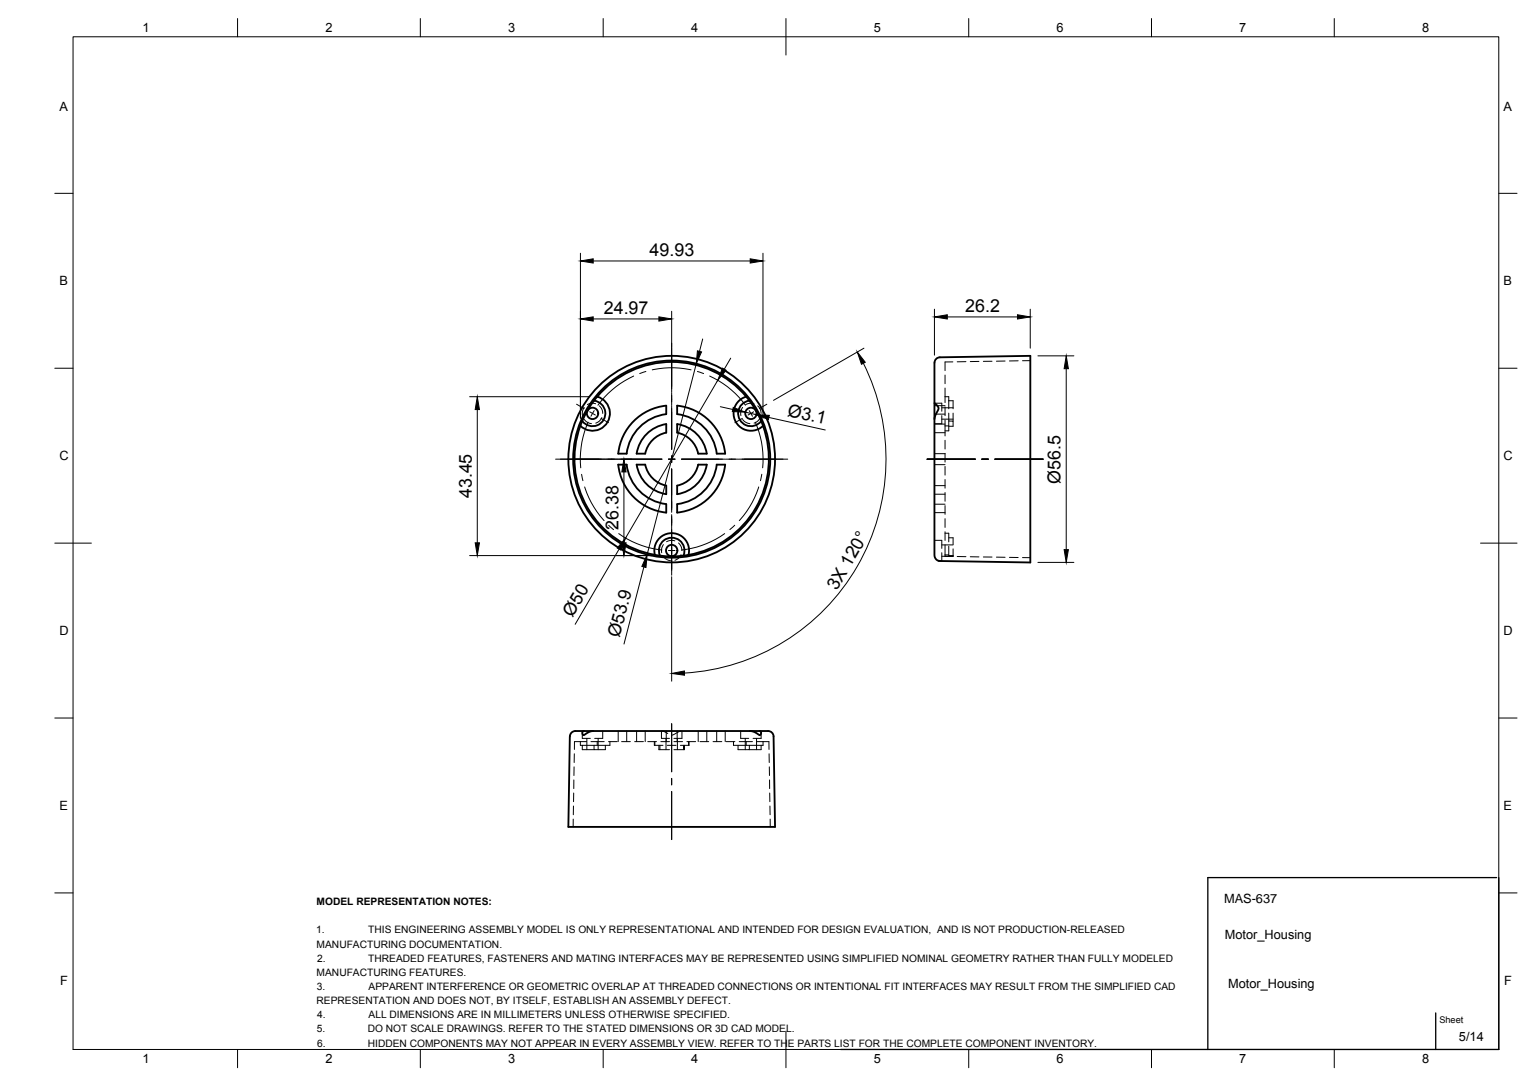
ISO-10303-21;
HEADER;
FILE_DESCRIPTION((''),'2;1');
FILE_NAME('Motor_Housing.step','2026-10-09T10:11:57-07:00',(''),(''),'','','');
FILE_SCHEMA (('AUTOMOTIVE_DESIGN { 1 0 10303 214 3 1 1 }'));
ENDSEC;
DATA;
#10=MECHANICAL_DESIGN_GEOMETRIC_PRESENTATION_REPRESENTATION('',(#125),#13510);
#95=SHAPE_REPRESENTATION_RELATIONSHIP('SRR','None',#13565,#110) ;
#110=ADVANCED_BREP_SHAPE_REPRESENTATION('',(#157),#13497) ;
#125=STYLED_ITEM('',(#13649),#157) ;
#157=MANIFOLD_SOLID_BREP('Body1',#7374) ;
#217=FACE_BOUND('',#1283,.T.) ;
#218=FACE_BOUND('',#1286,.T.) ;
#219=FACE_BOUND('',#1292,.T.) ;
#220=FACE_BOUND('',#1335,.T.) ;
#221=FACE_BOUND('',#1336,.T.) ;
#222=FACE_BOUND('',#1337,.T.) ;
#223=FACE_BOUND('',#1338,.T.) ;
#224=FACE_BOUND('',#1339,.T.) ;
#225=FACE_BOUND('',#1340,.T.) ;
#226=FACE_BOUND('',#1341,.T.) ;
#227=FACE_BOUND('',#1342,.T.) ;
#228=FACE_BOUND('',#1346,.T.) ;
#229=FACE_BOUND('',#1348,.T.) ;
#230=FACE_BOUND('',#1350,.T.) ;
#231=FACE_BOUND('',#1351,.T.) ;
#232=FACE_BOUND('',#1352,.T.) ;
#233=FACE_BOUND('',#1353,.T.) ;
#234=FACE_BOUND('',#1354,.T.) ;
#235=FACE_BOUND('',#1355,.T.) ;
#236=FACE_BOUND('',#1356,.T.) ;
#237=FACE_BOUND('',#1357,.T.) ;
#238=FACE_BOUND('',#1360,.T.) ;
#239=FACE_BOUND('',#1364,.T.) ;
#324=PLANE('',#7894) ;
#325=PLANE('',#7899) ;
#326=PLANE('',#7919) ;
#327=PLANE('',#7929) ;
#328=PLANE('',#7933) ;
#329=PLANE('',#7944) ;
#330=PLANE('',#7948) ;
#331=PLANE('',#7952) ;
#332=PLANE('',#7956) ;
#333=PLANE('',#7960) ;
#334=PLANE('',#7964) ;
#335=PLANE('',#7965) ;
#336=PLANE('',#7969) ;
#337=PLANE('',#7973) ;
#338=PLANE('',#7977) ;
#339=PLANE('',#7981) ;
#340=PLANE('',#7985) ;
#341=PLANE('',#7989) ;
#342=PLANE('',#7993) ;
#343=PLANE('',#7997) ;
#344=PLANE('',#8001) ;
#345=PLANE('',#8009) ;
#346=PLANE('',#8010) ;
#347=PLANE('',#8014) ;
#348=PLANE('',#8016) ;
#349=PLANE('',#8018) ;
#350=PLANE('',#8029) ;
#351=PLANE('',#8034) ;
#489=B_SPLINE_CURVE_WITH_KNOTS('',3,(#12264,#12265,#12266,#12267,#12268,
#12269,#12270,#12271,#12272,#12273,#12274,#12275,#12276,#12277,#12278,#12279,
#12280,#12281,#12282,#12283,#12284,#12285,#12286,#12287,#12288,#12289,#12290,
#12291,#12292,#12293,#12294,#12295,#12296,#12297),.UNSPECIFIED.,.F.,.F.,
(4,2,2,2,2,2,2,2,2,2,2,2,2,2,2,2,4),(0.531805899879346,0.536333824755711,
0.591897384336284,0.667209604638838,0.739839654066166,0.796834727976756,
0.805195853248504,0.808326840958196,0.810223650281403,0.812270988818894,
0.815029287812512,0.821153230725477,0.854786642673204,0.894100597636804,
0.968451976824404,1.02522403229621,1.04311608969068),.UNSPECIFIED.) ;
#490=B_SPLINE_CURVE_WITH_KNOTS('',3,(#12324,#12325,#12326,#12327,#12328,
#12329,#12330,#12331,#12332,#12333,#12334,#12335,#12336,#12337,#12338,#12339,
#12340,#12341,#12342,#12343,#12344,#12345,#12346,#12347,#12348,#12349,#12350,
#12351,#12352,#12353,#12354,#12355,#12356,#12357),.UNSPECIFIED.,.F.,.F.,
(4,2,2,2,2,2,2,2,2,2,2,2,2,2,2,2,4),(-1.04311608843254,-1.02522403109388,
-0.968451975747413,-0.894100596714524,-0.854786641825103,-0.821153229937673,
-0.815029287031212,-0.812270988041687,-0.810223649507742,-0.808326840188323,
-0.805195852486152,-0.796834727237095,-0.739839653424281,-0.667209604095289,
-0.591897383884855,-0.536333824369451,-0.531805899490485),.UNSPECIFIED.) ;
#491=B_SPLINE_CURVE_WITH_KNOTS('',3,(#12358,#12359,#12360,#12361,#12362,
#12363,#12364,#12365,#12366,#12367,#12368,#12369,#12370,#12371,#12372,#12373,
#12374,#12375,#12376,#12377,#12378,#12379,#12380,#12381,#12382,#12383,#12384,
#12385,#12386,#12387,#12388,#12389,#12390,#12391),.UNSPECIFIED.,.F.,.F.,
(4,2,2,2,2,2,2,2,2,2,2,2,2,2,2,2,4),(-1.04311608859891,-1.02522403125026,
-0.968451975875515,-0.8941005968091,-0.854786641903559,-0.821153230003261,
-0.815029287094133,-0.812270988104498,-0.8102236495713,-0.808326840252012,
-0.805195852547876,-0.796834727295025,-0.73983965345829,-0.667209604102352,
-0.59189738386758,-0.53633382433688,-0.531805899459014),.UNSPECIFIED.) ;
#497=TOROIDAL_SURFACE('',#8027,26.3501962679,1.5) ;
#601=CYLINDRICAL_SURFACE('',#7897,1.55) ;
#602=CYLINDRICAL_SURFACE('',#7902,26.5728722547) ;
#603=CYLINDRICAL_SURFACE('',#7906,3.5) ;
#604=CYLINDRICAL_SURFACE('',#7916,4.75) ;
#605=CYLINDRICAL_SURFACE('',#7923,3.5) ;
#606=CYLINDRICAL_SURFACE('',#7926,3.5) ;
#607=CYLINDRICAL_SURFACE('',#7937,4.75) ;
#608=CYLINDRICAL_SURFACE('',#7939,4.75) ;
#609=CYLINDRICAL_SURFACE('',#7941,12.4) ;
#610=CYLINDRICAL_SURFACE('',#7945,14.7) ;
#611=CYLINDRICAL_SURFACE('',#7949,7.4) ;
#612=CYLINDRICAL_SURFACE('',#7953,9.7) ;
#613=CYLINDRICAL_SURFACE('',#7957,12.4) ;
#614=CYLINDRICAL_SURFACE('',#7961,14.7) ;
#615=CYLINDRICAL_SURFACE('',#7966,12.4) ;
#616=CYLINDRICAL_SURFACE('',#7970,14.7) ;
#617=CYLINDRICAL_SURFACE('',#7974,9.7) ;
#618=CYLINDRICAL_SURFACE('',#7978,7.4) ;
#619=CYLINDRICAL_SURFACE('',#7982,9.7) ;
#620=CYLINDRICAL_SURFACE('',#7986,7.4) ;
#621=CYLINDRICAL_SURFACE('',#7990,7.4) ;
#622=CYLINDRICAL_SURFACE('',#7994,9.7) ;
#623=CYLINDRICAL_SURFACE('',#7998,14.7) ;
#624=CYLINDRICAL_SURFACE('',#8002,12.4) ;
#625=CYLINDRICAL_SURFACE('',#8005,26.5728722547) ;
#626=CYLINDRICAL_SURFACE('',#8007,26.5728722547) ;
#627=CYLINDRICAL_SURFACE('',#8011,2.8) ;
#628=CYLINDRICAL_SURFACE('',#8032,2.8) ;
#629=CYLINDRICAL_SURFACE('',#8033,1.55) ;
#630=CYLINDRICAL_SURFACE('',#8037,2.8) ;
#631=CYLINDRICAL_SURFACE('',#8038,1.55) ;
#804=FACE_OUTER_BOUND('',#1282,.T.) ;
#805=FACE_OUTER_BOUND('',#1284,.T.) ;
#806=FACE_OUTER_BOUND('',#1285,.T.) ;
#807=FACE_OUTER_BOUND('',#1287,.T.) ;
#808=FACE_OUTER_BOUND('',#1288,.T.) ;
#809=FACE_OUTER_BOUND('',#1289,.T.) ;
#810=FACE_OUTER_BOUND('',#1290,.T.) ;
#811=FACE_OUTER_BOUND('',#1291,.T.) ;
#812=FACE_OUTER_BOUND('',#1293,.T.) ;
#813=FACE_OUTER_BOUND('',#1294,.T.) ;
#814=FACE_OUTER_BOUND('',#1295,.T.) ;
#815=FACE_OUTER_BOUND('',#1296,.T.) ;
#816=FACE_OUTER_BOUND('',#1297,.T.) ;
#817=FACE_OUTER_BOUND('',#1298,.T.) ;
#818=FACE_OUTER_BOUND('',#1299,.T.) ;
#819=FACE_OUTER_BOUND('',#1300,.T.) ;
#820=FACE_OUTER_BOUND('',#1301,.T.) ;
#821=FACE_OUTER_BOUND('',#1302,.T.) ;
#822=FACE_OUTER_BOUND('',#1303,.T.) ;
#823=FACE_OUTER_BOUND('',#1304,.T.) ;
#824=FACE_OUTER_BOUND('',#1305,.T.) ;
#825=FACE_OUTER_BOUND('',#1306,.T.) ;
#826=FACE_OUTER_BOUND('',#1307,.T.) ;
#827=FACE_OUTER_BOUND('',#1308,.T.) ;
#828=FACE_OUTER_BOUND('',#1309,.T.) ;
#829=FACE_OUTER_BOUND('',#1310,.T.) ;
#830=FACE_OUTER_BOUND('',#1311,.T.) ;
#831=FACE_OUTER_BOUND('',#1312,.T.) ;
#832=FACE_OUTER_BOUND('',#1313,.T.) ;
#833=FACE_OUTER_BOUND('',#1314,.T.) ;
#834=FACE_OUTER_BOUND('',#1315,.T.) ;
#835=FACE_OUTER_BOUND('',#1316,.T.) ;
#836=FACE_OUTER_BOUND('',#1317,.T.) ;
#837=FACE_OUTER_BOUND('',#1318,.T.) ;
#838=FACE_OUTER_BOUND('',#1319,.T.) ;
#839=FACE_OUTER_BOUND('',#1320,.T.) ;
#840=FACE_OUTER_BOUND('',#1321,.T.) ;
#841=FACE_OUTER_BOUND('',#1322,.T.) ;
#842=FACE_OUTER_BOUND('',#1323,.T.) ;
#843=FACE_OUTER_BOUND('',#1324,.T.) ;
#844=FACE_OUTER_BOUND('',#1325,.T.) ;
#845=FACE_OUTER_BOUND('',#1326,.T.) ;
#846=FACE_OUTER_BOUND('',#1327,.T.) ;
#847=FACE_OUTER_BOUND('',#1328,.T.) ;
#848=FACE_OUTER_BOUND('',#1329,.T.) ;
#849=FACE_OUTER_BOUND('',#1330,.T.) ;
#850=FACE_OUTER_BOUND('',#1331,.T.) ;
#851=FACE_OUTER_BOUND('',#1332,.T.) ;
#852=FACE_OUTER_BOUND('',#1333,.T.) ;
#853=FACE_OUTER_BOUND('',#1334,.T.) ;
#854=FACE_OUTER_BOUND('',#1343,.T.) ;
#855=FACE_OUTER_BOUND('',#1344,.T.) ;
#856=FACE_OUTER_BOUND('',#1345,.T.) ;
#857=FACE_OUTER_BOUND('',#1347,.T.) ;
#858=FACE_OUTER_BOUND('',#1349,.T.) ;
#859=FACE_OUTER_BOUND('',#1358,.T.) ;
#860=FACE_OUTER_BOUND('',#1359,.T.) ;
#861=FACE_OUTER_BOUND('',#1361,.T.) ;
#862=FACE_OUTER_BOUND('',#1362,.T.) ;
#863=FACE_OUTER_BOUND('',#1363,.T.) ;
#864=FACE_OUTER_BOUND('',#1365,.T.) ;
#865=FACE_OUTER_BOUND('',#1366,.T.) ;
#1282=EDGE_LOOP('',(#5566)) ;
#1283=EDGE_LOOP('',(#5567)) ;
#1284=EDGE_LOOP('',(#5568,#5569,#5570,#5571)) ;
#1285=EDGE_LOOP('',(#5572,#5573)) ;
#1286=EDGE_LOOP('',(#5574)) ;
#1287=EDGE_LOOP('',(#5575,#5576,#5577,#5578,#5579,#5580,#5581,#5582)) ;
#1288=EDGE_LOOP('',(#5583,#5584,#5585,#5586)) ;
#1289=EDGE_LOOP('',(#5587,#5588,#5589,#5590,#5591,#5592,#5593,#5594,#5595,
#5596)) ;
#1290=EDGE_LOOP('',(#5597,#5598,#5599,#5600)) ;
#1291=EDGE_LOOP('',(#5601)) ;
#1292=EDGE_LOOP('',(#5602)) ;
#1293=EDGE_LOOP('',(#5603,#5604,#5605,#5606)) ;
#1294=EDGE_LOOP('',(#5607,#5608,#5609,#5610)) ;
#1295=EDGE_LOOP('',(#5611,#5612,#5613,#5614)) ;
#1296=EDGE_LOOP('',(#5615,#5616,#5617,#5618)) ;
#1297=EDGE_LOOP('',(#5619,#5620,#5621,#5622)) ;
#1298=EDGE_LOOP('',(#5623,#5624,#5625,#5626)) ;
#1299=EDGE_LOOP('',(#5627,#5628,#5629,#5630)) ;
#1300=EDGE_LOOP('',(#5631,#5632,#5633,#5634)) ;
#1301=EDGE_LOOP('',(#5635,#5636,#5637,#5638)) ;
#1302=EDGE_LOOP('',(#5639,#5640,#5641,#5642)) ;
#1303=EDGE_LOOP('',(#5643,#5644,#5645,#5646)) ;
#1304=EDGE_LOOP('',(#5647,#5648,#5649,#5650)) ;
#1305=EDGE_LOOP('',(#5651,#5652,#5653,#5654)) ;
#1306=EDGE_LOOP('',(#5655,#5656,#5657,#5658)) ;
#1307=EDGE_LOOP('',(#5659,#5660,#5661,#5662)) ;
#1308=EDGE_LOOP('',(#5663,#5664,#5665,#5666)) ;
#1309=EDGE_LOOP('',(#5667,#5668,#5669,#5670)) ;
#1310=EDGE_LOOP('',(#5671,#5672,#5673,#5674)) ;
#1311=EDGE_LOOP('',(#5675,#5676,#5677,#5678)) ;
#1312=EDGE_LOOP('',(#5679,#5680,#5681,#5682)) ;
#1313=EDGE_LOOP('',(#5683,#5684,#5685,#5686)) ;
#1314=EDGE_LOOP('',(#5687,#5688,#5689,#5690)) ;
#1315=EDGE_LOOP('',(#5691,#5692,#5693,#5694)) ;
#1316=EDGE_LOOP('',(#5695,#5696,#5697,#5698)) ;
#1317=EDGE_LOOP('',(#5699,#5700,#5701,#5702)) ;
#1318=EDGE_LOOP('',(#5703,#5704,#5705,#5706)) ;
#1319=EDGE_LOOP('',(#5707,#5708,#5709,#5710)) ;
#1320=EDGE_LOOP('',(#5711,#5712,#5713,#5714)) ;
#1321=EDGE_LOOP('',(#5715,#5716,#5717,#5718)) ;
#1322=EDGE_LOOP('',(#5719,#5720,#5721,#5722)) ;
#1323=EDGE_LOOP('',(#5723,#5724,#5725,#5726)) ;
#1324=EDGE_LOOP('',(#5727,#5728,#5729,#5730)) ;
#1325=EDGE_LOOP('',(#5731,#5732,#5733,#5734)) ;
#1326=EDGE_LOOP('',(#5735,#5736,#5737,#5738)) ;
#1327=EDGE_LOOP('',(#5739,#5740,#5741,#5742)) ;
#1328=EDGE_LOOP('',(#5743,#5744,#5745,#5746)) ;
#1329=EDGE_LOOP('',(#5747,#5748,#5749,#5750)) ;
#1330=EDGE_LOOP('',(#5751,#5752,#5753,#5754)) ;
#1331=EDGE_LOOP('',(#5755,#5756,#5757,#5758)) ;
#1332=EDGE_LOOP('',(#5759,#5760,#5761,#5762,#5763,#5764,#5765,#5766)) ;
#1333=EDGE_LOOP('',(#5767,#5768,#5769,#5770,#5771,#5772,#5773,#5774)) ;
#1334=EDGE_LOOP('',(#5775,#5776,#5777,#5778,#5779,#5780,#5781)) ;
#1335=EDGE_LOOP('',(#5782,#5783,#5784,#5785)) ;
#1336=EDGE_LOOP('',(#5786,#5787,#5788,#5789)) ;
#1337=EDGE_LOOP('',(#5790,#5791,#5792,#5793)) ;
#1338=EDGE_LOOP('',(#5794,#5795,#5796,#5797)) ;
#1339=EDGE_LOOP('',(#5798,#5799,#5800,#5801)) ;
#1340=EDGE_LOOP('',(#5802,#5803,#5804,#5805)) ;
#1341=EDGE_LOOP('',(#5806,#5807,#5808,#5809)) ;
#1342=EDGE_LOOP('',(#5810,#5811,#5812,#5813)) ;
#1343=EDGE_LOOP('',(#5814,#5815,#5816,#5817)) ;
#1344=EDGE_LOOP('',(#5818,#5819,#5820,#5821,#5822,#5823)) ;
#1345=EDGE_LOOP('',(#5824,#5825)) ;
#1346=EDGE_LOOP('',(#5826)) ;
#1347=EDGE_LOOP('',(#5827,#5828)) ;
#1348=EDGE_LOOP('',(#5829)) ;
#1349=EDGE_LOOP('',(#5830,#5831,#5832,#5833,#5834,#5835,#5836,#5837,#5838,
#5839)) ;
#1350=EDGE_LOOP('',(#5840,#5841,#5842,#5843)) ;
#1351=EDGE_LOOP('',(#5844,#5845,#5846,#5847)) ;
#1352=EDGE_LOOP('',(#5848,#5849,#5850,#5851)) ;
#1353=EDGE_LOOP('',(#5852,#5853,#5854,#5855)) ;
#1354=EDGE_LOOP('',(#5856,#5857,#5858,#5859)) ;
#1355=EDGE_LOOP('',(#5860,#5861,#5862,#5863)) ;
#1356=EDGE_LOOP('',(#5864,#5865,#5866,#5867)) ;
#1357=EDGE_LOOP('',(#5868,#5869,#5870,#5871)) ;
#1358=EDGE_LOOP('',(#5872,#5873,#5874,#5875,#5876,#5877,#5878,#5879,#5880,
#5881)) ;
#1359=EDGE_LOOP('',(#5882)) ;
#1360=EDGE_LOOP('',(#5883)) ;
#1361=EDGE_LOOP('',(#5884,#5885,#5886,#5887,#5888,#5889)) ;
#1362=EDGE_LOOP('',(#5890,#5891,#5892,#5893)) ;
#1363=EDGE_LOOP('',(#5894)) ;
#1364=EDGE_LOOP('',(#5895)) ;
#1365=EDGE_LOOP('',(#5896,#5897,#5898,#5899,#5900,#5901)) ;
#1366=EDGE_LOOP('',(#5902,#5903,#5904,#5905)) ;
#1822=LINE('',#11975,#2316) ;
#1823=LINE('',#11987,#2317) ;
#1824=LINE('',#11990,#2318) ;
#1825=LINE('',#11992,#2319) ;
#1826=LINE('',#11995,#2320) ;
#1827=LINE('',#12011,#2321) ;
#1828=LINE('',#12021,#2322) ;
#1829=LINE('',#12026,#2323) ;
#1830=LINE('',#12030,#2324) ;
#1831=LINE('',#12035,#2325) ;
#1832=LINE('',#12039,#2326) ;
#1833=LINE('',#12054,#2327) ;
#1834=LINE('',#12056,#2328) ;
#1835=LINE('',#12058,#2329) ;
#1836=LINE('',#12060,#2330) ;
#1837=LINE('',#12064,#2331) ;
#1838=LINE('',#12068,#2332) ;
#1839=LINE('',#12072,#2333) ;
#1840=LINE('',#12074,#2334) ;
#1841=LINE('',#12075,#2335) ;
#1842=LINE('',#12080,#2336) ;
#1843=LINE('',#12083,#2337) ;
#1844=LINE('',#12084,#2338) ;
#1845=LINE('',#12088,#2339) ;
#1846=LINE('',#12092,#2340) ;
#1847=LINE('',#12096,#2341) ;
#1848=LINE('',#12098,#2342) ;
#1849=LINE('',#12099,#2343) ;
#1850=LINE('',#12104,#2344) ;
#1851=LINE('',#12107,#2345) ;
#1852=LINE('',#12108,#2346) ;
#1853=LINE('',#12112,#2347) ;
#1854=LINE('',#12116,#2348) ;
#1855=LINE('',#12121,#2349) ;
#1856=LINE('',#12122,#2350) ;
#1857=LINE('',#12123,#2351) ;
#1858=LINE('',#12128,#2352) ;
#1859=LINE('',#12131,#2353) ;
#1860=LINE('',#12132,#2354) ;
#1861=LINE('',#12136,#2355) ;
#1862=LINE('',#12138,#2356) ;
#1863=LINE('',#12140,#2357) ;
#1864=LINE('',#12141,#2358) ;
#1865=LINE('',#12145,#2359) ;
#1866=LINE('',#12151,#2360) ;
#1867=LINE('',#12152,#2361) ;
#1868=LINE('',#12153,#2362) ;
#1869=LINE('',#12160,#2363) ;
#1870=LINE('',#12162,#2364) ;
#1871=LINE('',#12164,#2365) ;
#1872=LINE('',#12165,#2366) ;
#1873=LINE('',#12170,#2367) ;
#1874=LINE('',#12175,#2368) ;
#1875=LINE('',#12176,#2369) ;
#1876=LINE('',#12177,#2370) ;
#1877=LINE('',#12184,#2371) ;
#1878=LINE('',#12186,#2372) ;
#1879=LINE('',#12188,#2373) ;
#1880=LINE('',#12189,#2374) ;
#1881=LINE('',#12194,#2375) ;
#1882=LINE('',#12199,#2376) ;
#1883=LINE('',#12200,#2377) ;
#1884=LINE('',#12201,#2378) ;
#1885=LINE('',#12208,#2379) ;
#1886=LINE('',#12210,#2380) ;
#1887=LINE('',#12212,#2381) ;
#1888=LINE('',#12213,#2382) ;
#1889=LINE('',#12217,#2383) ;
#1890=LINE('',#12223,#2384) ;
#1891=LINE('',#12224,#2385) ;
#1892=LINE('',#12225,#2386) ;
#1893=LINE('',#12232,#2387) ;
#1894=LINE('',#12234,#2388) ;
#1895=LINE('',#12236,#2389) ;
#1896=LINE('',#12237,#2390) ;
#1897=LINE('',#12242,#2391) ;
#1898=LINE('',#12247,#2392) ;
#1899=LINE('',#12248,#2393) ;
#1900=LINE('',#12249,#2394) ;
#1901=LINE('',#12299,#2395) ;
#1902=LINE('',#12398,#2396) ;
#1903=LINE('',#12400,#2397) ;
#1904=LINE('',#12407,#2398) ;
#1905=LINE('',#12409,#2399) ;
#2316=VECTOR('',#9396,1.55) ;
#2317=VECTOR('',#9409,1.) ;
#2318=VECTOR('',#9412,1.) ;
#2319=VECTOR('',#9413,1.) ;
#2320=VECTOR('',#9416,1.) ;
#2321=VECTOR('',#9435,26.5728722547) ;
#2322=VECTOR('',#9450,27.85) ;
#2323=VECTOR('',#9455,1.) ;
#2324=VECTOR('',#9458,1.) ;
#2325=VECTOR('',#9463,1.) ;
#2326=VECTOR('',#9466,1.) ;
#2327=VECTOR('',#9487,1.) ;
#2328=VECTOR('',#9490,1.) ;
#2329=VECTOR('',#9493,1.) ;
#2330=VECTOR('',#9496,1.) ;
#2331=VECTOR('',#9499,1.) ;
#2332=VECTOR('',#9502,1.) ;
#2333=VECTOR('',#9507,1.) ;
#2334=VECTOR('',#9508,1.) ;
#2335=VECTOR('',#9509,1.) ;
#2336=VECTOR('',#9514,1.) ;
#2337=VECTOR('',#9519,1.) ;
#2338=VECTOR('',#9520,1.) ;
#2339=VECTOR('',#9523,1.) ;
#2340=VECTOR('',#9526,1.) ;
#2341=VECTOR('',#9531,1.) ;
#2342=VECTOR('',#9532,1.) ;
#2343=VECTOR('',#9533,1.) ;
#2344=VECTOR('',#9538,1.) ;
#2345=VECTOR('',#9543,1.) ;
#2346=VECTOR('',#9544,1.) ;
#2347=VECTOR('',#9547,1.) ;
#2348=VECTOR('',#9550,1.) ;
#2349=VECTOR('',#9555,1.) ;
#2350=VECTOR('',#9556,1.) ;
#2351=VECTOR('',#9557,1.) ;
#2352=VECTOR('',#9562,1.) ;
#2353=VECTOR('',#9567,1.) ;
#2354=VECTOR('',#9568,1.) ;
#2355=VECTOR('',#9571,1.) ;
#2356=VECTOR('',#9572,1.) ;
#2357=VECTOR('',#9573,1.) ;
#2358=VECTOR('',#9574,1.) ;
#2359=VECTOR('',#9577,1.) ;
#2360=VECTOR('',#9584,1.) ;
#2361=VECTOR('',#9585,1.) ;
#2362=VECTOR('',#9586,1.) ;
#2363=VECTOR('',#9595,1.) ;
#2364=VECTOR('',#9596,1.) ;
#2365=VECTOR('',#9597,1.) ;
#2366=VECTOR('',#9598,1.) ;
#2367=VECTOR('',#9603,1.) ;
#2368=VECTOR('',#9608,1.) ;
#2369=VECTOR('',#9609,1.) ;
#2370=VECTOR('',#9610,1.) ;
#2371=VECTOR('',#9619,1.) ;
#2372=VECTOR('',#9620,1.) ;
#2373=VECTOR('',#9621,1.) ;
#2374=VECTOR('',#9622,1.) ;
#2375=VECTOR('',#9627,1.) ;
#2376=VECTOR('',#9632,1.) ;
#2377=VECTOR('',#9633,1.) ;
#2378=VECTOR('',#9634,1.) ;
#2379=VECTOR('',#9643,1.) ;
#2380=VECTOR('',#9644,1.) ;
#2381=VECTOR('',#9645,1.) ;
#2382=VECTOR('',#9646,1.) ;
#2383=VECTOR('',#9649,1.) ;
#2384=VECTOR('',#9656,1.) ;
#2385=VECTOR('',#9657,1.) ;
#2386=VECTOR('',#9658,1.) ;
#2387=VECTOR('',#9667,1.) ;
#2388=VECTOR('',#9668,1.) ;
#2389=VECTOR('',#9669,1.) ;
#2390=VECTOR('',#9670,1.) ;
#2391=VECTOR('',#9675,1.) ;
#2392=VECTOR('',#9680,1.) ;
#2393=VECTOR('',#9681,1.) ;
#2394=VECTOR('',#9682,1.) ;
#2395=VECTOR('',#9707,2.8) ;
#2396=VECTOR('',#9746,2.8) ;
#2397=VECTOR('',#9749,1.55) ;
#2398=VECTOR('',#9758,2.8) ;
#2399=VECTOR('',#9761,1.55) ;
#2815=CIRCLE('',#7895,2.8) ;
#2816=CIRCLE('',#7896,1.55) ;
#2817=CIRCLE('',#7898,1.55) ;
#2818=CIRCLE('',#7900,26.5728722547) ;
#2819=CIRCLE('',#7901,3.5) ;
#2820=CIRCLE('',#7903,26.5728722547) ;
#2821=CIRCLE('',#7904,26.5728722547) ;
#2822=CIRCLE('',#7905,26.5728722547) ;
#2823=CIRCLE('',#7907,3.5) ;
#2824=CIRCLE('',#7909,26.5728722547) ;
#2825=CIRCLE('',#7910,26.5728722547) ;
#2826=CIRCLE('',#7911,26.5728722547) ;
#2827=CIRCLE('',#7912,26.5728722547) ;
#2828=CIRCLE('',#7913,26.5728722547) ;
#2829=CIRCLE('',#7914,26.5728722547) ;
#2830=CIRCLE('',#7915,26.9498298789) ;
#2831=CIRCLE('',#7917,4.75) ;
#2832=CIRCLE('',#7918,4.75) ;
#2833=CIRCLE('',#7920,28.25) ;
#2834=CIRCLE('',#7922,27.85) ;
#2835=CIRCLE('',#7924,3.5) ;
#2836=CIRCLE('',#7925,3.5) ;
#2837=CIRCLE('',#7927,3.5) ;
#2838=CIRCLE('',#7928,3.5) ;
#2839=CIRCLE('',#7930,26.5728722547) ;
#2840=CIRCLE('',#7931,4.75) ;
#2841=CIRCLE('',#7932,26.5728722547) ;
#2842=CIRCLE('',#7934,26.5728722547) ;
#2843=CIRCLE('',#7935,4.75) ;
#2844=CIRCLE('',#7936,26.5728722547) ;
#2845=CIRCLE('',#7938,4.75) ;
#2846=CIRCLE('',#7940,4.75) ;
#2847=CIRCLE('',#7942,12.4) ;
#2848=CIRCLE('',#7943,12.4) ;
#2849=CIRCLE('',#7946,14.7) ;
#2850=CIRCLE('',#7947,14.7) ;
#2851=CIRCLE('',#7950,7.4) ;
#2852=CIRCLE('',#7951,7.4) ;
#2853=CIRCLE('',#7954,9.7) ;
#2854=CIRCLE('',#7955,9.7) ;
#2855=CIRCLE('',#7958,12.4) ;
#2856=CIRCLE('',#7959,12.4) ;
#2857=CIRCLE('',#7962,14.7) ;
#2858=CIRCLE('',#7963,14.7) ;
#2859=CIRCLE('',#7967,12.4) ;
#2860=CIRCLE('',#7968,12.4) ;
#2861=CIRCLE('',#7971,14.7) ;
#2862=CIRCLE('',#7972,14.7) ;
#2863=CIRCLE('',#7975,9.7) ;
#2864=CIRCLE('',#7976,9.7) ;
#2865=CIRCLE('',#7979,7.4) ;
#2866=CIRCLE('',#7980,7.4) ;
#2867=CIRCLE('',#7983,9.7) ;
#2868=CIRCLE('',#7984,9.7) ;
#2869=CIRCLE('',#7987,7.4) ;
#2870=CIRCLE('',#7988,7.4) ;
#2871=CIRCLE('',#7991,7.4) ;
#2872=CIRCLE('',#7992,7.4) ;
#2873=CIRCLE('',#7995,9.7) ;
#2874=CIRCLE('',#7996,9.7) ;
#2875=CIRCLE('',#7999,14.7) ;
#2876=CIRCLE('',#8000,14.7) ;
#2877=CIRCLE('',#8003,12.4) ;
#2878=CIRCLE('',#8004,12.4) ;
#2879=CIRCLE('',#8006,26.5728722547) ;
#2880=CIRCLE('',#8008,26.5728722547) ;
#2881=CIRCLE('',#8012,2.8) ;
#2882=CIRCLE('',#8013,2.8) ;
#2883=CIRCLE('',#8015,1.55) ;
#2884=CIRCLE('',#8017,1.55) ;
#2885=CIRCLE('',#8019,2.8) ;
#2886=CIRCLE('',#8020,2.8) ;
#2887=CIRCLE('',#8021,26.3501962679) ;
#2888=CIRCLE('',#8022,26.3501962679) ;
#2889=CIRCLE('',#8023,2.8) ;
#2890=CIRCLE('',#8024,2.8) ;
#2891=CIRCLE('',#8025,26.3501962679) ;
#2892=CIRCLE('',#8026,26.3501962679) ;
#2893=CIRCLE('',#8028,1.5) ;
#2894=CIRCLE('',#8030,2.8) ;
#2895=CIRCLE('',#8031,1.55) ;
#2896=CIRCLE('',#8035,2.8) ;
#2897=CIRCLE('',#8036,1.55) ;
#3385=VERTEX_POINT('',#11969) ;
#3386=VERTEX_POINT('',#11971) ;
#3387=VERTEX_POINT('',#11974) ;
#3388=VERTEX_POINT('',#11978) ;
#3389=VERTEX_POINT('',#11979) ;
#3390=VERTEX_POINT('',#11983) ;
#3391=VERTEX_POINT('',#11984) ;
#3392=VERTEX_POINT('',#11986) ;
#3393=VERTEX_POINT('',#11988) ;
#3394=VERTEX_POINT('',#11991) ;
#3395=VERTEX_POINT('',#11993) ;
#3396=VERTEX_POINT('',#11999) ;
#3397=VERTEX_POINT('',#12000) ;
#3398=VERTEX_POINT('',#12002) ;
#3399=VERTEX_POINT('',#12005) ;
#3400=VERTEX_POINT('',#12007) ;
#3401=VERTEX_POINT('',#12010) ;
#3402=VERTEX_POINT('',#12017) ;
#3403=VERTEX_POINT('',#12020) ;
#3404=VERTEX_POINT('',#12024) ;
#3405=VERTEX_POINT('',#12025) ;
#3406=VERTEX_POINT('',#12027) ;
#3407=VERTEX_POINT('',#12029) ;
#3408=VERTEX_POINT('',#12033) ;
#3409=VERTEX_POINT('',#12034) ;
#3410=VERTEX_POINT('',#12036) ;
#3411=VERTEX_POINT('',#12038) ;
#3412=VERTEX_POINT('',#12042) ;
#3413=VERTEX_POINT('',#12044) ;
#3414=VERTEX_POINT('',#12048) ;
#3415=VERTEX_POINT('',#12050) ;
#3416=VERTEX_POINT('',#12062) ;
#3417=VERTEX_POINT('',#12063) ;
#3418=VERTEX_POINT('',#12065) ;
#3419=VERTEX_POINT('',#12067) ;
#3420=VERTEX_POINT('',#12071) ;
#3421=VERTEX_POINT('',#12073) ;
#3422=VERTEX_POINT('',#12077) ;
#3423=VERTEX_POINT('',#12079) ;
#3424=VERTEX_POINT('',#12086) ;
#3425=VERTEX_POINT('',#12087) ;
#3426=VERTEX_POINT('',#12089) ;
#3427=VERTEX_POINT('',#12091) ;
#3428=VERTEX_POINT('',#12095) ;
#3429=VERTEX_POINT('',#12097) ;
#3430=VERTEX_POINT('',#12101) ;
#3431=VERTEX_POINT('',#12103) ;
#3432=VERTEX_POINT('',#12110) ;
#3433=VERTEX_POINT('',#12111) ;
#3434=VERTEX_POINT('',#12113) ;
#3435=VERTEX_POINT('',#12115) ;
#3436=VERTEX_POINT('',#12119) ;
#3437=VERTEX_POINT('',#12120) ;
#3438=VERTEX_POINT('',#12125) ;
#3439=VERTEX_POINT('',#12127) ;
#3440=VERTEX_POINT('',#12134) ;
#3441=VERTEX_POINT('',#12135) ;
#3442=VERTEX_POINT('',#12137) ;
#3443=VERTEX_POINT('',#12139) ;
#3444=VERTEX_POINT('',#12143) ;
#3445=VERTEX_POINT('',#12144) ;
#3446=VERTEX_POINT('',#12149) ;
#3447=VERTEX_POINT('',#12150) ;
#3448=VERTEX_POINT('',#12158) ;
#3449=VERTEX_POINT('',#12159) ;
#3450=VERTEX_POINT('',#12161) ;
#3451=VERTEX_POINT('',#12163) ;
#3452=VERTEX_POINT('',#12167) ;
#3453=VERTEX_POINT('',#12169) ;
#3454=VERTEX_POINT('',#12173) ;
#3455=VERTEX_POINT('',#12174) ;
#3456=VERTEX_POINT('',#12182) ;
#3457=VERTEX_POINT('',#12183) ;
#3458=VERTEX_POINT('',#12185) ;
#3459=VERTEX_POINT('',#12187) ;
#3460=VERTEX_POINT('',#12191) ;
#3461=VERTEX_POINT('',#12193) ;
#3462=VERTEX_POINT('',#12197) ;
#3463=VERTEX_POINT('',#12198) ;
#3464=VERTEX_POINT('',#12206) ;
#3465=VERTEX_POINT('',#12207) ;
#3466=VERTEX_POINT('',#12209) ;
#3467=VERTEX_POINT('',#12211) ;
#3468=VERTEX_POINT('',#12215) ;
#3469=VERTEX_POINT('',#12216) ;
#3470=VERTEX_POINT('',#12221) ;
#3471=VERTEX_POINT('',#12222) ;
#3472=VERTEX_POINT('',#12230) ;
#3473=VERTEX_POINT('',#12231) ;
#3474=VERTEX_POINT('',#12233) ;
#3475=VERTEX_POINT('',#12235) ;
#3476=VERTEX_POINT('',#12239) ;
#3477=VERTEX_POINT('',#12241) ;
#3478=VERTEX_POINT('',#12245) ;
#3479=VERTEX_POINT('',#12246) ;
#3480=VERTEX_POINT('',#12260) ;
#3481=VERTEX_POINT('',#12261) ;
#3482=VERTEX_POINT('',#12263) ;
#3483=VERTEX_POINT('',#12301) ;
#3484=VERTEX_POINT('',#12304) ;
#3485=VERTEX_POINT('',#12307) ;
#3486=VERTEX_POINT('',#12308) ;
#3487=VERTEX_POINT('',#12310) ;
#3488=VERTEX_POINT('',#12313) ;
#3489=VERTEX_POINT('',#12315) ;
#3490=VERTEX_POINT('',#12317) ;
#3491=VERTEX_POINT('',#12319) ;
#3492=VERTEX_POINT('',#12393) ;
#3493=VERTEX_POINT('',#12395) ;
#3494=VERTEX_POINT('',#12402) ;
#3495=VERTEX_POINT('',#12404) ;
#4170=EDGE_CURVE('',#3385,#3385,#2815,.T.) ;
#4171=EDGE_CURVE('',#3386,#3386,#2816,.T.) ;
#4172=EDGE_CURVE('',#3386,#3387,#1822,.T.) ;
#4173=EDGE_CURVE('',#3387,#3387,#2817,.T.) ;
#4174=EDGE_CURVE('',#3388,#3389,#2818,.T.) ;
#4175=EDGE_CURVE('',#3389,#3388,#2819,.T.) ;
#4176=EDGE_CURVE('',#3390,#3391,#2820,.T.) ;
#4177=EDGE_CURVE('',#3391,#3392,#1823,.T.) ;
#4178=EDGE_CURVE('',#3393,#3392,#2821,.T.) ;
#4179=EDGE_CURVE('',#3393,#3389,#1824,.T.) ;
#4180=EDGE_CURVE('',#3394,#3388,#1825,.T.) ;
#4181=EDGE_CURVE('',#3395,#3394,#2822,.T.) ;
#4182=EDGE_CURVE('',#3390,#3395,#1826,.T.) ;
#4183=EDGE_CURVE('',#3393,#3394,#2823,.T.) ;
#4184=EDGE_CURVE('',#3396,#3397,#2824,.T.) ;
#4185=EDGE_CURVE('',#3398,#3396,#2825,.T.) ;
#4186=EDGE_CURVE('',#3391,#3398,#2826,.T.) ;
#4187=EDGE_CURVE('',#3399,#3390,#2827,.T.) ;
#4188=EDGE_CURVE('',#3400,#3399,#2828,.T.) ;
#4189=EDGE_CURVE('',#3397,#3400,#2829,.T.) ;
#4190=EDGE_CURVE('',#3397,#3401,#1827,.T.) ;
#4191=EDGE_CURVE('',#3401,#3401,#2830,.T.) ;
#4192=EDGE_CURVE('',#3391,#3390,#2831,.T.) ;
#4193=EDGE_CURVE('',#3392,#3395,#2832,.T.) ;
#4194=EDGE_CURVE('',#3402,#3402,#2833,.T.) ;
#4195=EDGE_CURVE('',#3402,#3403,#1828,.T.) ;
#4196=EDGE_CURVE('',#3403,#3403,#2834,.T.) ;
#4197=EDGE_CURVE('',#3404,#3405,#1829,.T.) ;
#4198=EDGE_CURVE('',#3406,#3405,#2835,.T.) ;
#4199=EDGE_CURVE('',#3407,#3406,#1830,.T.) ;
#4200=EDGE_CURVE('',#3407,#3404,#2836,.T.) ;
#4201=EDGE_CURVE('',#3408,#3409,#1831,.T.) ;
#4202=EDGE_CURVE('',#3410,#3409,#2837,.T.) ;
#4203=EDGE_CURVE('',#3411,#3410,#1832,.T.) ;
#4204=EDGE_CURVE('',#3411,#3408,#2838,.T.) ;
#4205=EDGE_CURVE('',#3411,#3412,#2839,.T.) ;
#4206=EDGE_CURVE('',#3412,#3413,#2840,.T.) ;
#4207=EDGE_CURVE('',#3413,#3408,#2841,.T.) ;
#4208=EDGE_CURVE('',#3407,#3414,#2842,.T.) ;
#4209=EDGE_CURVE('',#3414,#3415,#2843,.T.) ;
#4210=EDGE_CURVE('',#3415,#3404,#2844,.T.) ;
#4211=EDGE_CURVE('',#3396,#3412,#1833,.T.) ;
#4212=EDGE_CURVE('',#3396,#3398,#2845,.T.) ;
#4213=EDGE_CURVE('',#3398,#3413,#1834,.T.) ;
#4214=EDGE_CURVE('',#3399,#3414,#1835,.T.) ;
#4215=EDGE_CURVE('',#3399,#3400,#2846,.T.) ;
#4216=EDGE_CURVE('',#3400,#3415,#1836,.T.) ;
#4217=EDGE_CURVE('',#3416,#3417,#1837,.F.) ;
#4218=EDGE_CURVE('',#3416,#3418,#2847,.F.) ;
#4219=EDGE_CURVE('',#3418,#3419,#1838,.F.) ;
#4220=EDGE_CURVE('',#3417,#3419,#2848,.F.) ;
#4221=EDGE_CURVE('',#3417,#3420,#1839,.T.) ;
#4222=EDGE_CURVE('',#3421,#3420,#1840,.T.) ;
#4223=EDGE_CURVE('',#3421,#3416,#1841,.F.) ;
#4224=EDGE_CURVE('',#3420,#3422,#2849,.F.) ;
#4225=EDGE_CURVE('',#3423,#3422,#1842,.F.) ;
#4226=EDGE_CURVE('',#3423,#3421,#2850,.T.) ;
#4227=EDGE_CURVE('',#3422,#3419,#1843,.T.) ;
#4228=EDGE_CURVE('',#3418,#3423,#1844,.F.) ;
#4229=EDGE_CURVE('',#3424,#3425,#1845,.F.) ;
#4230=EDGE_CURVE('',#3424,#3426,#2851,.F.) ;
#4231=EDGE_CURVE('',#3426,#3427,#1846,.F.) ;
#4232=EDGE_CURVE('',#3425,#3427,#2852,.F.) ;
#4233=EDGE_CURVE('',#3425,#3428,#1847,.T.) ;
#4234=EDGE_CURVE('',#3429,#3428,#1848,.T.) ;
#4235=EDGE_CURVE('',#3429,#3424,#1849,.F.) ;
#4236=EDGE_CURVE('',#3428,#3430,#2853,.F.) ;
#4237=EDGE_CURVE('',#3431,#3430,#1850,.F.) ;
#4238=EDGE_CURVE('',#3431,#3429,#2854,.T.) ;
#4239=EDGE_CURVE('',#3430,#3427,#1851,.T.) ;
#4240=EDGE_CURVE('',#3426,#3431,#1852,.F.) ;
#4241=EDGE_CURVE('',#3432,#3433,#1853,.F.) ;
#4242=EDGE_CURVE('',#3432,#3434,#2855,.F.) ;
#4243=EDGE_CURVE('',#3434,#3435,#1854,.F.) ;
#4244=EDGE_CURVE('',#3433,#3435,#2856,.F.) ;
#4245=EDGE_CURVE('',#3436,#3437,#1855,.T.) ;
#4246=EDGE_CURVE('',#3436,#3432,#1856,.T.) ;
#4247=EDGE_CURVE('',#3437,#3433,#1857,.T.) ;
#4248=EDGE_CURVE('',#3437,#3438,#2857,.F.) ;
#4249=EDGE_CURVE('',#3439,#3438,#1858,.F.) ;
#4250=EDGE_CURVE('',#3439,#3436,#2858,.T.) ;
#4251=EDGE_CURVE('',#3438,#3435,#1859,.T.) ;
#4252=EDGE_CURVE('',#3434,#3439,#1860,.F.) ;
#4253=EDGE_CURVE('',#3440,#3441,#1861,.T.) ;
#4254=EDGE_CURVE('',#3440,#3442,#1862,.T.) ;
#4255=EDGE_CURVE('',#3442,#3443,#1863,.T.) ;
#4256=EDGE_CURVE('',#3441,#3443,#1864,.T.) ;
#4257=EDGE_CURVE('',#3444,#3445,#1865,.F.) ;
#4258=EDGE_CURVE('',#3444,#3440,#2859,.F.) ;
#4259=EDGE_CURVE('',#3445,#3441,#2860,.F.) ;
#4260=EDGE_CURVE('',#3446,#3447,#1866,.T.) ;
#4261=EDGE_CURVE('',#3446,#3444,#1867,.T.) ;
#4262=EDGE_CURVE('',#3447,#3445,#1868,.T.) ;
#4263=EDGE_CURVE('',#3447,#3443,#2861,.F.) ;
#4264=EDGE_CURVE('',#3442,#3446,#2862,.T.) ;
#4265=EDGE_CURVE('',#3448,#3449,#1869,.T.) ;
#4266=EDGE_CURVE('',#3450,#3449,#1870,.T.) ;
#4267=EDGE_CURVE('',#3450,#3451,#1871,.F.) ;
#4268=EDGE_CURVE('',#3451,#3448,#1872,.T.) ;
#4269=EDGE_CURVE('',#3449,#3452,#2863,.F.) ;
#4270=EDGE_CURVE('',#3453,#3452,#1873,.F.) ;
#4271=EDGE_CURVE('',#3453,#3450,#2864,.T.) ;
#4272=EDGE_CURVE('',#3454,#3455,#1874,.T.) ;
#4273=EDGE_CURVE('',#3454,#3453,#1875,.T.) ;
#4274=EDGE_CURVE('',#3455,#3452,#1876,.T.) ;
#4275=EDGE_CURVE('',#3451,#3454,#2865,.F.) ;
#4276=EDGE_CURVE('',#3448,#3455,#2866,.F.) ;
#4277=EDGE_CURVE('',#3456,#3457,#1877,.T.) ;
#4278=EDGE_CURVE('',#3456,#3458,#1878,.T.) ;
#4279=EDGE_CURVE('',#3458,#3459,#1879,.T.) ;
#4280=EDGE_CURVE('',#3457,#3459,#1880,.T.) ;
#4281=EDGE_CURVE('',#3457,#3460,#2867,.F.) ;
#4282=EDGE_CURVE('',#3461,#3460,#1881,.F.) ;
#4283=EDGE_CURVE('',#3461,#3456,#2868,.T.) ;
#4284=EDGE_CURVE('',#3462,#3463,#1882,.T.) ;
#4285=EDGE_CURVE('',#3462,#3461,#1883,.T.) ;
#4286=EDGE_CURVE('',#3463,#3460,#1884,.T.) ;
#4287=EDGE_CURVE('',#3458,#3462,#2869,.F.) ;
#4288=EDGE_CURVE('',#3459,#3463,#2870,.F.) ;
#4289=EDGE_CURVE('',#3464,#3465,#1885,.T.) ;
#4290=EDGE_CURVE('',#3466,#3465,#1886,.T.) ;
#4291=EDGE_CURVE('',#3466,#3467,#1887,.F.) ;
#4292=EDGE_CURVE('',#3467,#3464,#1888,.T.) ;
#4293=EDGE_CURVE('',#3468,#3469,#1889,.F.) ;
#4294=EDGE_CURVE('',#3468,#3466,#2871,.F.) ;
#4295=EDGE_CURVE('',#3469,#3465,#2872,.F.) ;
#4296=EDGE_CURVE('',#3470,#3471,#1890,.T.) ;
#4297=EDGE_CURVE('',#3470,#3468,#1891,.T.) ;
#4298=EDGE_CURVE('',#3471,#3469,#1892,.T.) ;
#4299=EDGE_CURVE('',#3471,#3464,#2873,.F.) ;
#4300=EDGE_CURVE('',#3467,#3470,#2874,.T.) ;
#4301=EDGE_CURVE('',#3472,#3473,#1893,.T.) ;
#4302=EDGE_CURVE('',#3474,#3473,#1894,.T.) ;
#4303=EDGE_CURVE('',#3474,#3475,#1895,.F.) ;
#4304=EDGE_CURVE('',#3475,#3472,#1896,.T.) ;
#4305=EDGE_CURVE('',#3473,#3476,#2875,.F.) ;
#4306=EDGE_CURVE('',#3477,#3476,#1897,.F.) ;
#4307=EDGE_CURVE('',#3477,#3474,#2876,.T.) ;
#4308=EDGE_CURVE('',#3478,#3479,#1898,.T.) ;
#4309=EDGE_CURVE('',#3478,#3477,#1899,.T.) ;
#4310=EDGE_CURVE('',#3479,#3476,#1900,.T.) ;
#4311=EDGE_CURVE('',#3475,#3478,#2877,.F.) ;
#4312=EDGE_CURVE('',#3472,#3479,#2878,.F.) ;
#4313=EDGE_CURVE('',#3409,#3410,#2879,.T.) ;
#4314=EDGE_CURVE('',#3405,#3406,#2880,.T.) ;
#4315=EDGE_CURVE('',#3480,#3481,#2881,.T.) ;
#4316=EDGE_CURVE('',#3482,#3480,#489,.F.) ;
#4317=EDGE_CURVE('',#3481,#3482,#2882,.T.) ;
#4318=EDGE_CURVE('',#3481,#3385,#1901,.T.) ;
#4319=EDGE_CURVE('',#3483,#3483,#2883,.T.) ;
#4320=EDGE_CURVE('',#3484,#3484,#2884,.T.) ;
#4321=EDGE_CURVE('',#3485,#3486,#2885,.T.) ;
#4322=EDGE_CURVE('',#3486,#3487,#2886,.T.) ;
#4323=EDGE_CURVE('',#3480,#3487,#2887,.T.) ;
#4324=EDGE_CURVE('',#3488,#3482,#2888,.T.) ;
#4325=EDGE_CURVE('',#3488,#3489,#2889,.T.) ;
#4326=EDGE_CURVE('',#3489,#3490,#2890,.T.) ;
#4327=EDGE_CURVE('',#3491,#3490,#2891,.T.) ;
#4328=EDGE_CURVE('',#3485,#3491,#2892,.T.) ;
#4329=EDGE_CURVE('',#3403,#3491,#2893,.T.) ;
#4330=EDGE_CURVE('',#3488,#3490,#490,.F.) ;
#4331=EDGE_CURVE('',#3485,#3487,#491,.F.) ;
#4332=EDGE_CURVE('',#3492,#3492,#2894,.T.) ;
#4333=EDGE_CURVE('',#3493,#3493,#2895,.T.) ;
#4334=EDGE_CURVE('',#3489,#3492,#1902,.T.) ;
#4335=EDGE_CURVE('',#3493,#3483,#1903,.T.) ;
#4336=EDGE_CURVE('',#3494,#3494,#2896,.T.) ;
#4337=EDGE_CURVE('',#3495,#3495,#2897,.T.) ;
#4338=EDGE_CURVE('',#3486,#3494,#1904,.T.) ;
#4339=EDGE_CURVE('',#3495,#3484,#1905,.T.) ;
#5566=ORIENTED_EDGE('',*,*,#4170,.F.) ;
#5567=ORIENTED_EDGE('',*,*,#4171,.T.) ;
#5568=ORIENTED_EDGE('',*,*,#4171,.F.) ;
#5569=ORIENTED_EDGE('',*,*,#4172,.T.) ;
#5570=ORIENTED_EDGE('',*,*,#4173,.T.) ;
#5571=ORIENTED_EDGE('',*,*,#4172,.F.) ;
#5572=ORIENTED_EDGE('',*,*,#4174,.T.) ;
#5573=ORIENTED_EDGE('',*,*,#4175,.T.) ;
#5574=ORIENTED_EDGE('',*,*,#4173,.F.) ;
#5575=ORIENTED_EDGE('',*,*,#4176,.T.) ;
#5576=ORIENTED_EDGE('',*,*,#4177,.T.) ;
#5577=ORIENTED_EDGE('',*,*,#4178,.F.) ;
#5578=ORIENTED_EDGE('',*,*,#4179,.T.) ;
#5579=ORIENTED_EDGE('',*,*,#4174,.F.) ;
#5580=ORIENTED_EDGE('',*,*,#4180,.F.) ;
#5581=ORIENTED_EDGE('',*,*,#4181,.F.) ;
#5582=ORIENTED_EDGE('',*,*,#4182,.F.) ;
#5583=ORIENTED_EDGE('',*,*,#4180,.T.) ;
#5584=ORIENTED_EDGE('',*,*,#4175,.F.) ;
#5585=ORIENTED_EDGE('',*,*,#4179,.F.) ;
#5586=ORIENTED_EDGE('',*,*,#4183,.T.) ;
#5587=ORIENTED_EDGE('',*,*,#4184,.F.) ;
#5588=ORIENTED_EDGE('',*,*,#4185,.F.) ;
#5589=ORIENTED_EDGE('',*,*,#4186,.F.) ;
#5590=ORIENTED_EDGE('',*,*,#4176,.F.) ;
#5591=ORIENTED_EDGE('',*,*,#4187,.F.) ;
#5592=ORIENTED_EDGE('',*,*,#4188,.F.) ;
#5593=ORIENTED_EDGE('',*,*,#4189,.F.) ;
#5594=ORIENTED_EDGE('',*,*,#4190,.T.) ;
#5595=ORIENTED_EDGE('',*,*,#4191,.T.) ;
#5596=ORIENTED_EDGE('',*,*,#4190,.F.) ;
#5597=ORIENTED_EDGE('',*,*,#4177,.F.) ;
#5598=ORIENTED_EDGE('',*,*,#4192,.T.) ;
#5599=ORIENTED_EDGE('',*,*,#4182,.T.) ;
#5600=ORIENTED_EDGE('',*,*,#4193,.F.) ;
#5601=ORIENTED_EDGE('',*,*,#4194,.T.) ;
#5602=ORIENTED_EDGE('',*,*,#4191,.F.) ;
#5603=ORIENTED_EDGE('',*,*,#4194,.F.) ;
#5604=ORIENTED_EDGE('',*,*,#4195,.T.) ;
#5605=ORIENTED_EDGE('',*,*,#4196,.T.) ;
#5606=ORIENTED_EDGE('',*,*,#4195,.F.) ;
#5607=ORIENTED_EDGE('',*,*,#4197,.T.) ;
#5608=ORIENTED_EDGE('',*,*,#4198,.F.) ;
#5609=ORIENTED_EDGE('',*,*,#4199,.F.) ;
#5610=ORIENTED_EDGE('',*,*,#4200,.T.) ;
#5611=ORIENTED_EDGE('',*,*,#4201,.T.) ;
#5612=ORIENTED_EDGE('',*,*,#4202,.F.) ;
#5613=ORIENTED_EDGE('',*,*,#4203,.F.) ;
#5614=ORIENTED_EDGE('',*,*,#4204,.T.) ;
#5615=ORIENTED_EDGE('',*,*,#4205,.T.) ;
#5616=ORIENTED_EDGE('',*,*,#4206,.T.) ;
#5617=ORIENTED_EDGE('',*,*,#4207,.T.) ;
#5618=ORIENTED_EDGE('',*,*,#4204,.F.) ;
#5619=ORIENTED_EDGE('',*,*,#4208,.T.) ;
#5620=ORIENTED_EDGE('',*,*,#4209,.T.) ;
#5621=ORIENTED_EDGE('',*,*,#4210,.T.) ;
#5622=ORIENTED_EDGE('',*,*,#4200,.F.) ;
#5623=ORIENTED_EDGE('',*,*,#4211,.F.) ;
#5624=ORIENTED_EDGE('',*,*,#4212,.T.) ;
#5625=ORIENTED_EDGE('',*,*,#4213,.T.) ;
#5626=ORIENTED_EDGE('',*,*,#4206,.F.) ;
#5627=ORIENTED_EDGE('',*,*,#4214,.F.) ;
#5628=ORIENTED_EDGE('',*,*,#4215,.T.) ;
#5629=ORIENTED_EDGE('',*,*,#4216,.T.) ;
#5630=ORIENTED_EDGE('',*,*,#4209,.F.) ;
#5631=ORIENTED_EDGE('',*,*,#4217,.F.) ;
#5632=ORIENTED_EDGE('',*,*,#4218,.T.) ;
#5633=ORIENTED_EDGE('',*,*,#4219,.T.) ;
#5634=ORIENTED_EDGE('',*,*,#4220,.F.) ;
#5635=ORIENTED_EDGE('',*,*,#4221,.T.) ;
#5636=ORIENTED_EDGE('',*,*,#4222,.F.) ;
#5637=ORIENTED_EDGE('',*,*,#4223,.T.) ;
#5638=ORIENTED_EDGE('',*,*,#4217,.T.) ;
#5639=ORIENTED_EDGE('',*,*,#4224,.T.) ;
#5640=ORIENTED_EDGE('',*,*,#4225,.F.) ;
#5641=ORIENTED_EDGE('',*,*,#4226,.T.) ;
#5642=ORIENTED_EDGE('',*,*,#4222,.T.) ;
#5643=ORIENTED_EDGE('',*,*,#4227,.T.) ;
#5644=ORIENTED_EDGE('',*,*,#4219,.F.) ;
#5645=ORIENTED_EDGE('',*,*,#4228,.T.) ;
#5646=ORIENTED_EDGE('',*,*,#4225,.T.) ;
#5647=ORIENTED_EDGE('',*,*,#4229,.F.) ;
#5648=ORIENTED_EDGE('',*,*,#4230,.T.) ;
#5649=ORIENTED_EDGE('',*,*,#4231,.T.) ;
#5650=ORIENTED_EDGE('',*,*,#4232,.F.) ;
#5651=ORIENTED_EDGE('',*,*,#4233,.T.) ;
#5652=ORIENTED_EDGE('',*,*,#4234,.F.) ;
#5653=ORIENTED_EDGE('',*,*,#4235,.T.) ;
#5654=ORIENTED_EDGE('',*,*,#4229,.T.) ;
#5655=ORIENTED_EDGE('',*,*,#4236,.T.) ;
#5656=ORIENTED_EDGE('',*,*,#4237,.F.) ;
#5657=ORIENTED_EDGE('',*,*,#4238,.T.) ;
#5658=ORIENTED_EDGE('',*,*,#4234,.T.) ;
#5659=ORIENTED_EDGE('',*,*,#4239,.T.) ;
#5660=ORIENTED_EDGE('',*,*,#4231,.F.) ;
#5661=ORIENTED_EDGE('',*,*,#4240,.T.) ;
#5662=ORIENTED_EDGE('',*,*,#4237,.T.) ;
#5663=ORIENTED_EDGE('',*,*,#4241,.F.) ;
#5664=ORIENTED_EDGE('',*,*,#4242,.T.) ;
#5665=ORIENTED_EDGE('',*,*,#4243,.T.) ;
#5666=ORIENTED_EDGE('',*,*,#4244,.F.) ;
#5667=ORIENTED_EDGE('',*,*,#4245,.F.) ;
#5668=ORIENTED_EDGE('',*,*,#4246,.T.) ;
#5669=ORIENTED_EDGE('',*,*,#4241,.T.) ;
#5670=ORIENTED_EDGE('',*,*,#4247,.F.) ;
#5671=ORIENTED_EDGE('',*,*,#4248,.T.) ;
#5672=ORIENTED_EDGE('',*,*,#4249,.F.) ;
#5673=ORIENTED_EDGE('',*,*,#4250,.T.) ;
#5674=ORIENTED_EDGE('',*,*,#4245,.T.) ;
#5675=ORIENTED_EDGE('',*,*,#4251,.T.) ;
#5676=ORIENTED_EDGE('',*,*,#4243,.F.) ;
#5677=ORIENTED_EDGE('',*,*,#4252,.T.) ;
#5678=ORIENTED_EDGE('',*,*,#4249,.T.) ;
#5679=ORIENTED_EDGE('',*,*,#4253,.F.) ;
#5680=ORIENTED_EDGE('',*,*,#4254,.T.) ;
#5681=ORIENTED_EDGE('',*,*,#4255,.T.) ;
#5682=ORIENTED_EDGE('',*,*,#4256,.F.) ;
#5683=ORIENTED_EDGE('',*,*,#4257,.F.) ;
#5684=ORIENTED_EDGE('',*,*,#4258,.T.) ;
#5685=ORIENTED_EDGE('',*,*,#4253,.T.) ;
#5686=ORIENTED_EDGE('',*,*,#4259,.F.) ;
#5687=ORIENTED_EDGE('',*,*,#4260,.F.) ;
#5688=ORIENTED_EDGE('',*,*,#4261,.T.) ;
#5689=ORIENTED_EDGE('',*,*,#4257,.T.) ;
#5690=ORIENTED_EDGE('',*,*,#4262,.F.) ;
#5691=ORIENTED_EDGE('',*,*,#4263,.T.) ;
#5692=ORIENTED_EDGE('',*,*,#4255,.F.) ;
#5693=ORIENTED_EDGE('',*,*,#4264,.T.) ;
#5694=ORIENTED_EDGE('',*,*,#4260,.T.) ;
#5695=ORIENTED_EDGE('',*,*,#4265,.T.) ;
#5696=ORIENTED_EDGE('',*,*,#4266,.F.) ;
#5697=ORIENTED_EDGE('',*,*,#4267,.T.) ;
#5698=ORIENTED_EDGE('',*,*,#4268,.T.) ;
#5699=ORIENTED_EDGE('',*,*,#4269,.T.) ;
#5700=ORIENTED_EDGE('',*,*,#4270,.F.) ;
#5701=ORIENTED_EDGE('',*,*,#4271,.T.) ;
#5702=ORIENTED_EDGE('',*,*,#4266,.T.) ;
#5703=ORIENTED_EDGE('',*,*,#4272,.F.) ;
#5704=ORIENTED_EDGE('',*,*,#4273,.T.) ;
#5705=ORIENTED_EDGE('',*,*,#4270,.T.) ;
#5706=ORIENTED_EDGE('',*,*,#4274,.F.) ;
#5707=ORIENTED_EDGE('',*,*,#4268,.F.) ;
#5708=ORIENTED_EDGE('',*,*,#4275,.T.) ;
#5709=ORIENTED_EDGE('',*,*,#4272,.T.) ;
#5710=ORIENTED_EDGE('',*,*,#4276,.F.) ;
#5711=ORIENTED_EDGE('',*,*,#4277,.F.) ;
#5712=ORIENTED_EDGE('',*,*,#4278,.T.) ;
#5713=ORIENTED_EDGE('',*,*,#4279,.T.) ;
#5714=ORIENTED_EDGE('',*,*,#4280,.F.) ;
#5715=ORIENTED_EDGE('',*,*,#4281,.T.) ;
#5716=ORIENTED_EDGE('',*,*,#4282,.F.) ;
#5717=ORIENTED_EDGE('',*,*,#4283,.T.) ;
#5718=ORIENTED_EDGE('',*,*,#4277,.T.) ;
#5719=ORIENTED_EDGE('',*,*,#4284,.F.) ;
#5720=ORIENTED_EDGE('',*,*,#4285,.T.) ;
#5721=ORIENTED_EDGE('',*,*,#4282,.T.) ;
#5722=ORIENTED_EDGE('',*,*,#4286,.F.) ;
#5723=ORIENTED_EDGE('',*,*,#4279,.F.) ;
#5724=ORIENTED_EDGE('',*,*,#4287,.T.) ;
#5725=ORIENTED_EDGE('',*,*,#4284,.T.) ;
#5726=ORIENTED_EDGE('',*,*,#4288,.F.) ;
#5727=ORIENTED_EDGE('',*,*,#4289,.T.) ;
#5728=ORIENTED_EDGE('',*,*,#4290,.F.) ;
#5729=ORIENTED_EDGE('',*,*,#4291,.T.) ;
#5730=ORIENTED_EDGE('',*,*,#4292,.T.) ;
#5731=ORIENTED_EDGE('',*,*,#4293,.F.) ;
#5732=ORIENTED_EDGE('',*,*,#4294,.T.) ;
#5733=ORIENTED_EDGE('',*,*,#4290,.T.) ;
#5734=ORIENTED_EDGE('',*,*,#4295,.F.) ;
#5735=ORIENTED_EDGE('',*,*,#4296,.F.) ;
#5736=ORIENTED_EDGE('',*,*,#4297,.T.) ;
#5737=ORIENTED_EDGE('',*,*,#4293,.T.) ;
#5738=ORIENTED_EDGE('',*,*,#4298,.F.) ;
#5739=ORIENTED_EDGE('',*,*,#4299,.T.) ;
#5740=ORIENTED_EDGE('',*,*,#4292,.F.) ;
#5741=ORIENTED_EDGE('',*,*,#4300,.T.) ;
#5742=ORIENTED_EDGE('',*,*,#4296,.T.) ;
#5743=ORIENTED_EDGE('',*,*,#4301,.T.) ;
#5744=ORIENTED_EDGE('',*,*,#4302,.F.) ;
#5745=ORIENTED_EDGE('',*,*,#4303,.T.) ;
#5746=ORIENTED_EDGE('',*,*,#4304,.T.) ;
#5747=ORIENTED_EDGE('',*,*,#4305,.T.) ;
#5748=ORIENTED_EDGE('',*,*,#4306,.F.) ;
#5749=ORIENTED_EDGE('',*,*,#4307,.T.) ;
#5750=ORIENTED_EDGE('',*,*,#4302,.T.) ;
#5751=ORIENTED_EDGE('',*,*,#4308,.F.) ;
#5752=ORIENTED_EDGE('',*,*,#4309,.T.) ;
#5753=ORIENTED_EDGE('',*,*,#4306,.T.) ;
#5754=ORIENTED_EDGE('',*,*,#4310,.F.) ;
#5755=ORIENTED_EDGE('',*,*,#4304,.F.) ;
#5756=ORIENTED_EDGE('',*,*,#4311,.T.) ;
#5757=ORIENTED_EDGE('',*,*,#4308,.T.) ;
#5758=ORIENTED_EDGE('',*,*,#4312,.F.) ;
#5759=ORIENTED_EDGE('',*,*,#4203,.T.) ;
#5760=ORIENTED_EDGE('',*,*,#4313,.F.) ;
#5761=ORIENTED_EDGE('',*,*,#4201,.F.) ;
#5762=ORIENTED_EDGE('',*,*,#4207,.F.) ;
#5763=ORIENTED_EDGE('',*,*,#4213,.F.) ;
#5764=ORIENTED_EDGE('',*,*,#4185,.T.) ;
#5765=ORIENTED_EDGE('',*,*,#4211,.T.) ;
#5766=ORIENTED_EDGE('',*,*,#4205,.F.) ;
#5767=ORIENTED_EDGE('',*,*,#4210,.F.) ;
#5768=ORIENTED_EDGE('',*,*,#4216,.F.) ;
#5769=ORIENTED_EDGE('',*,*,#4188,.T.) ;
#5770=ORIENTED_EDGE('',*,*,#4214,.T.) ;
#5771=ORIENTED_EDGE('',*,*,#4208,.F.) ;
#5772=ORIENTED_EDGE('',*,*,#4199,.T.) ;
#5773=ORIENTED_EDGE('',*,*,#4314,.F.) ;
#5774=ORIENTED_EDGE('',*,*,#4197,.F.) ;
#5775=ORIENTED_EDGE('',*,*,#4184,.T.) ;
#5776=ORIENTED_EDGE('',*,*,#4189,.T.) ;
#5777=ORIENTED_EDGE('',*,*,#4215,.F.) ;
#5778=ORIENTED_EDGE('',*,*,#4187,.T.) ;
#5779=ORIENTED_EDGE('',*,*,#4192,.F.) ;
#5780=ORIENTED_EDGE('',*,*,#4186,.T.) ;
#5781=ORIENTED_EDGE('',*,*,#4212,.F.) ;
#5782=ORIENTED_EDGE('',*,*,#4312,.T.) ;
#5783=ORIENTED_EDGE('',*,*,#4310,.T.) ;
#5784=ORIENTED_EDGE('',*,*,#4305,.F.) ;
#5785=ORIENTED_EDGE('',*,*,#4301,.F.) ;
#5786=ORIENTED_EDGE('',*,*,#4299,.F.) ;
#5787=ORIENTED_EDGE('',*,*,#4298,.T.) ;
#5788=ORIENTED_EDGE('',*,*,#4295,.T.) ;
#5789=ORIENTED_EDGE('',*,*,#4289,.F.) ;
#5790=ORIENTED_EDGE('',*,*,#4288,.T.) ;
#5791=ORIENTED_EDGE('',*,*,#4286,.T.) ;
#5792=ORIENTED_EDGE('',*,*,#4281,.F.) ;
#5793=ORIENTED_EDGE('',*,*,#4280,.T.) ;
#5794=ORIENTED_EDGE('',*,*,#4276,.T.) ;
#5795=ORIENTED_EDGE('',*,*,#4274,.T.) ;
#5796=ORIENTED_EDGE('',*,*,#4269,.F.) ;
#5797=ORIENTED_EDGE('',*,*,#4265,.F.) ;
#5798=ORIENTED_EDGE('',*,*,#4263,.F.) ;
#5799=ORIENTED_EDGE('',*,*,#4262,.T.) ;
#5800=ORIENTED_EDGE('',*,*,#4259,.T.) ;
#5801=ORIENTED_EDGE('',*,*,#4256,.T.) ;
#5802=ORIENTED_EDGE('',*,*,#4251,.F.) ;
#5803=ORIENTED_EDGE('',*,*,#4248,.F.) ;
#5804=ORIENTED_EDGE('',*,*,#4247,.T.) ;
#5805=ORIENTED_EDGE('',*,*,#4244,.T.) ;
#5806=ORIENTED_EDGE('',*,*,#4239,.F.) ;
#5807=ORIENTED_EDGE('',*,*,#4236,.F.) ;
#5808=ORIENTED_EDGE('',*,*,#4233,.F.) ;
#5809=ORIENTED_EDGE('',*,*,#4232,.T.) ;
#5810=ORIENTED_EDGE('',*,*,#4227,.F.) ;
#5811=ORIENTED_EDGE('',*,*,#4224,.F.) ;
#5812=ORIENTED_EDGE('',*,*,#4221,.F.) ;
#5813=ORIENTED_EDGE('',*,*,#4220,.T.) ;
#5814=ORIENTED_EDGE('',*,*,#4178,.T.) ;
#5815=ORIENTED_EDGE('',*,*,#4193,.T.) ;
#5816=ORIENTED_EDGE('',*,*,#4181,.T.) ;
#5817=ORIENTED_EDGE('',*,*,#4183,.F.) ;
#5818=ORIENTED_EDGE('',*,*,#4315,.F.) ;
#5819=ORIENTED_EDGE('',*,*,#4316,.F.) ;
#5820=ORIENTED_EDGE('',*,*,#4317,.F.) ;
#5821=ORIENTED_EDGE('',*,*,#4318,.T.) ;
#5822=ORIENTED_EDGE('',*,*,#4170,.T.) ;
#5823=ORIENTED_EDGE('',*,*,#4318,.F.) ;
#5824=ORIENTED_EDGE('',*,*,#4314,.T.) ;
#5825=ORIENTED_EDGE('',*,*,#4198,.T.) ;
#5826=ORIENTED_EDGE('',*,*,#4319,.F.) ;
#5827=ORIENTED_EDGE('',*,*,#4313,.T.) ;
#5828=ORIENTED_EDGE('',*,*,#4202,.T.) ;
#5829=ORIENTED_EDGE('',*,*,#4320,.F.) ;
#5830=ORIENTED_EDGE('',*,*,#4321,.T.) ;
#5831=ORIENTED_EDGE('',*,*,#4322,.T.) ;
#5832=ORIENTED_EDGE('',*,*,#4323,.F.) ;
#5833=ORIENTED_EDGE('',*,*,#4315,.T.) ;
#5834=ORIENTED_EDGE('',*,*,#4317,.T.) ;
#5835=ORIENTED_EDGE('',*,*,#4324,.F.) ;
#5836=ORIENTED_EDGE('',*,*,#4325,.T.) ;
#5837=ORIENTED_EDGE('',*,*,#4326,.T.) ;
#5838=ORIENTED_EDGE('',*,*,#4327,.F.) ;
#5839=ORIENTED_EDGE('',*,*,#4328,.F.) ;
#5840=ORIENTED_EDGE('',*,*,#4303,.F.) ;
#5841=ORIENTED_EDGE('',*,*,#4307,.F.) ;
#5842=ORIENTED_EDGE('',*,*,#4309,.F.) ;
#5843=ORIENTED_EDGE('',*,*,#4311,.F.) ;
#5844=ORIENTED_EDGE('',*,*,#4291,.F.) ;
#5845=ORIENTED_EDGE('',*,*,#4294,.F.) ;
#5846=ORIENTED_EDGE('',*,*,#4297,.F.) ;
#5847=ORIENTED_EDGE('',*,*,#4300,.F.) ;
#5848=ORIENTED_EDGE('',*,*,#4278,.F.) ;
#5849=ORIENTED_EDGE('',*,*,#4283,.F.) ;
#5850=ORIENTED_EDGE('',*,*,#4285,.F.) ;
#5851=ORIENTED_EDGE('',*,*,#4287,.F.) ;
#5852=ORIENTED_EDGE('',*,*,#4267,.F.) ;
#5853=ORIENTED_EDGE('',*,*,#4271,.F.) ;
#5854=ORIENTED_EDGE('',*,*,#4273,.F.) ;
#5855=ORIENTED_EDGE('',*,*,#4275,.F.) ;
#5856=ORIENTED_EDGE('',*,*,#4254,.F.) ;
#5857=ORIENTED_EDGE('',*,*,#4258,.F.) ;
#5858=ORIENTED_EDGE('',*,*,#4261,.F.) ;
#5859=ORIENTED_EDGE('',*,*,#4264,.F.) ;
#5860=ORIENTED_EDGE('',*,*,#4242,.F.) ;
#5861=ORIENTED_EDGE('',*,*,#4246,.F.) ;
#5862=ORIENTED_EDGE('',*,*,#4250,.F.) ;
#5863=ORIENTED_EDGE('',*,*,#4252,.F.) ;
#5864=ORIENTED_EDGE('',*,*,#4230,.F.) ;
#5865=ORIENTED_EDGE('',*,*,#4235,.F.) ;
#5866=ORIENTED_EDGE('',*,*,#4238,.F.) ;
#5867=ORIENTED_EDGE('',*,*,#4240,.F.) ;
#5868=ORIENTED_EDGE('',*,*,#4218,.F.) ;
#5869=ORIENTED_EDGE('',*,*,#4223,.F.) ;
#5870=ORIENTED_EDGE('',*,*,#4226,.F.) ;
#5871=ORIENTED_EDGE('',*,*,#4228,.F.) ;
#5872=ORIENTED_EDGE('',*,*,#4196,.F.) ;
#5873=ORIENTED_EDGE('',*,*,#4329,.T.) ;
#5874=ORIENTED_EDGE('',*,*,#4327,.T.) ;
#5875=ORIENTED_EDGE('',*,*,#4330,.F.) ;
#5876=ORIENTED_EDGE('',*,*,#4324,.T.) ;
#5877=ORIENTED_EDGE('',*,*,#4316,.T.) ;
#5878=ORIENTED_EDGE('',*,*,#4323,.T.) ;
#5879=ORIENTED_EDGE('',*,*,#4331,.F.) ;
#5880=ORIENTED_EDGE('',*,*,#4328,.T.) ;
#5881=ORIENTED_EDGE('',*,*,#4329,.F.) ;
#5882=ORIENTED_EDGE('',*,*,#4332,.F.) ;
#5883=ORIENTED_EDGE('',*,*,#4333,.T.) ;
#5884=ORIENTED_EDGE('',*,*,#4325,.F.) ;
#5885=ORIENTED_EDGE('',*,*,#4330,.T.) ;
#5886=ORIENTED_EDGE('',*,*,#4326,.F.) ;
#5887=ORIENTED_EDGE('',*,*,#4334,.T.) ;
#5888=ORIENTED_EDGE('',*,*,#4332,.T.) ;
#5889=ORIENTED_EDGE('',*,*,#4334,.F.) ;
#5890=ORIENTED_EDGE('',*,*,#4333,.F.) ;
#5891=ORIENTED_EDGE('',*,*,#4335,.T.) ;
#5892=ORIENTED_EDGE('',*,*,#4319,.T.) ;
#5893=ORIENTED_EDGE('',*,*,#4335,.F.) ;
#5894=ORIENTED_EDGE('',*,*,#4336,.F.) ;
#5895=ORIENTED_EDGE('',*,*,#4337,.T.) ;
#5896=ORIENTED_EDGE('',*,*,#4321,.F.) ;
#5897=ORIENTED_EDGE('',*,*,#4331,.T.) ;
#5898=ORIENTED_EDGE('',*,*,#4322,.F.) ;
#5899=ORIENTED_EDGE('',*,*,#4338,.T.) ;
#5900=ORIENTED_EDGE('',*,*,#4336,.T.) ;
#5901=ORIENTED_EDGE('',*,*,#4338,.F.) ;
#5902=ORIENTED_EDGE('',*,*,#4337,.F.) ;
#5903=ORIENTED_EDGE('',*,*,#4339,.T.) ;
#5904=ORIENTED_EDGE('',*,*,#4320,.T.) ;
#5905=ORIENTED_EDGE('',*,*,#4339,.F.) ;
#6883=CONICAL_SURFACE('',#7908,26.5728722547,0.0161770275042) ;
#6884=CONICAL_SURFACE('',#7921,27.85,0.0161770275042) ;
#7054=ADVANCED_FACE('',(#804,#217),#324,.F.) ;
#7055=ADVANCED_FACE('',(#805),#601,.F.) ;
#7056=ADVANCED_FACE('',(#806,#218),#325,.T.) ;
#7057=ADVANCED_FACE('',(#807),#602,.T.) ;
#7058=ADVANCED_FACE('',(#808),#603,.T.) ;
#7059=ADVANCED_FACE('',(#809),#6883,.F.) ;
#7060=ADVANCED_FACE('',(#810),#604,.T.) ;
#7061=ADVANCED_FACE('',(#811,#219),#326,.T.) ;
#7062=ADVANCED_FACE('',(#812),#6884,.T.) ;
#7063=ADVANCED_FACE('',(#813),#605,.T.) ;
#7064=ADVANCED_FACE('',(#814),#606,.T.) ;
#7065=ADVANCED_FACE('',(#815),#327,.T.) ;
#7066=ADVANCED_FACE('',(#816),#328,.T.) ;
#7067=ADVANCED_FACE('',(#817),#607,.T.) ;
#7068=ADVANCED_FACE('',(#818),#608,.T.) ;
#7069=ADVANCED_FACE('',(#819),#609,.T.) ;
#7070=ADVANCED_FACE('',(#820),#329,.F.) ;
#7071=ADVANCED_FACE('',(#821),#610,.F.) ;
#7072=ADVANCED_FACE('',(#822),#330,.F.) ;
#7073=ADVANCED_FACE('',(#823),#611,.T.) ;
#7074=ADVANCED_FACE('',(#824),#331,.F.) ;
#7075=ADVANCED_FACE('',(#825),#612,.F.) ;
#7076=ADVANCED_FACE('',(#826),#332,.F.) ;
#7077=ADVANCED_FACE('',(#827),#613,.T.) ;
#7078=ADVANCED_FACE('',(#828),#333,.T.) ;
#7079=ADVANCED_FACE('',(#829),#614,.F.) ;
#7080=ADVANCED_FACE('',(#830),#334,.F.) ;
#7081=ADVANCED_FACE('',(#831),#335,.T.) ;
#7082=ADVANCED_FACE('',(#832),#615,.T.) ;
#7083=ADVANCED_FACE('',(#833),#336,.T.) ;
#7084=ADVANCED_FACE('',(#834),#616,.F.) ;
#7085=ADVANCED_FACE('',(#835),#337,.F.) ;
#7086=ADVANCED_FACE('',(#836),#617,.F.) ;
#7087=ADVANCED_FACE('',(#837),#338,.T.) ;
#7088=ADVANCED_FACE('',(#838),#618,.T.) ;
#7089=ADVANCED_FACE('',(#839),#339,.T.) ;
#7090=ADVANCED_FACE('',(#840),#619,.F.) ;
#7091=ADVANCED_FACE('',(#841),#340,.T.) ;
#7092=ADVANCED_FACE('',(#842),#620,.T.) ;
#7093=ADVANCED_FACE('',(#843),#341,.F.) ;
#7094=ADVANCED_FACE('',(#844),#621,.T.) ;
#7095=ADVANCED_FACE('',(#845),#342,.T.) ;
#7096=ADVANCED_FACE('',(#846),#622,.F.) ;
#7097=ADVANCED_FACE('',(#847),#343,.F.) ;
#7098=ADVANCED_FACE('',(#848),#623,.F.) ;
#7099=ADVANCED_FACE('',(#849),#344,.T.) ;
#7100=ADVANCED_FACE('',(#850),#624,.T.) ;
#7101=ADVANCED_FACE('',(#851),#625,.T.) ;
#7102=ADVANCED_FACE('',(#852),#626,.T.) ;
#7103=ADVANCED_FACE('',(#853,#220,#221,#222,#223,#224,#225,#226,#227),#345,
 .T.) ;
#7104=ADVANCED_FACE('',(#854),#346,.T.) ;
#7105=ADVANCED_FACE('',(#855),#627,.F.) ;
#7106=ADVANCED_FACE('',(#856,#228),#347,.T.) ;
#7107=ADVANCED_FACE('',(#857,#229),#348,.T.) ;
#7108=ADVANCED_FACE('',(#858,#230,#231,#232,#233,#234,#235,#236,#237),#349,
 .F.) ;
#7109=ADVANCED_FACE('',(#859),#497,.T.) ;
#7110=ADVANCED_FACE('',(#860,#238),#350,.F.) ;
#7111=ADVANCED_FACE('',(#861),#628,.F.) ;
#7112=ADVANCED_FACE('',(#862),#629,.F.) ;
#7113=ADVANCED_FACE('',(#863,#239),#351,.F.) ;
#7114=ADVANCED_FACE('',(#864),#630,.F.) ;
#7115=ADVANCED_FACE('',(#865),#631,.F.) ;
#7374=CLOSED_SHELL('',(#7054,#7055,#7056,#7057,#7058,#7059,#7060,#7061,
#7062,#7063,#7064,#7065,#7066,#7067,#7068,#7069,#7070,#7071,#7072,#7073,
#7074,#7075,#7076,#7077,#7078,#7079,#7080,#7081,#7082,#7083,#7084,#7085,
#7086,#7087,#7088,#7089,#7090,#7091,#7092,#7093,#7094,#7095,#7096,#7097,
#7098,#7099,#7100,#7101,#7102,#7103,#7104,#7105,#7106,#7107,#7108,#7109,
#7110,#7111,#7112,#7113,#7114,#7115)) ;
#7893=AXIS2_PLACEMENT_3D('',#11967,#9386,#9387) ;
#7894=AXIS2_PLACEMENT_3D('',#11968,#9388,#9389) ;
#7895=AXIS2_PLACEMENT_3D('',#11970,#9390,#9391) ;
#7896=AXIS2_PLACEMENT_3D('',#11972,#9392,#9393) ;
#7897=AXIS2_PLACEMENT_3D('',#11973,#9394,#9395) ;
#7898=AXIS2_PLACEMENT_3D('',#11976,#9397,#9398) ;
#7899=AXIS2_PLACEMENT_3D('',#11977,#9399,#9400) ;
#7900=AXIS2_PLACEMENT_3D('',#11980,#9401,#9402) ;
#7901=AXIS2_PLACEMENT_3D('',#11981,#9403,#9404) ;
#7902=AXIS2_PLACEMENT_3D('',#11982,#9405,#9406) ;
#7903=AXIS2_PLACEMENT_3D('',#11985,#9407,#9408) ;
#7904=AXIS2_PLACEMENT_3D('',#11989,#9410,#9411) ;
#7905=AXIS2_PLACEMENT_3D('',#11994,#9414,#9415) ;
#7906=AXIS2_PLACEMENT_3D('',#11996,#9417,#9418) ;
#7907=AXIS2_PLACEMENT_3D('',#11997,#9419,#9420) ;
#7908=AXIS2_PLACEMENT_3D('',#11998,#9421,#9422) ;
#7909=AXIS2_PLACEMENT_3D('',#12001,#9423,#9424) ;
#7910=AXIS2_PLACEMENT_3D('',#12003,#9425,#9426) ;
#7911=AXIS2_PLACEMENT_3D('',#12004,#9427,#9428) ;
#7912=AXIS2_PLACEMENT_3D('',#12006,#9429,#9430) ;
#7913=AXIS2_PLACEMENT_3D('',#12008,#9431,#9432) ;
#7914=AXIS2_PLACEMENT_3D('',#12009,#9433,#9434) ;
#7915=AXIS2_PLACEMENT_3D('',#12012,#9436,#9437) ;
#7916=AXIS2_PLACEMENT_3D('',#12013,#9438,#9439) ;
#7917=AXIS2_PLACEMENT_3D('',#12014,#9440,#9441) ;
#7918=AXIS2_PLACEMENT_3D('',#12015,#9442,#9443) ;
#7919=AXIS2_PLACEMENT_3D('',#12016,#9444,#9445) ;
#7920=AXIS2_PLACEMENT_3D('',#12018,#9446,#9447) ;
#7921=AXIS2_PLACEMENT_3D('',#12019,#9448,#9449) ;
#7922=AXIS2_PLACEMENT_3D('',#12022,#9451,#9452) ;
#7923=AXIS2_PLACEMENT_3D('',#12023,#9453,#9454) ;
#7924=AXIS2_PLACEMENT_3D('',#12028,#9456,#9457) ;
#7925=AXIS2_PLACEMENT_3D('',#12031,#9459,#9460) ;
#7926=AXIS2_PLACEMENT_3D('',#12032,#9461,#9462) ;
#7927=AXIS2_PLACEMENT_3D('',#12037,#9464,#9465) ;
#7928=AXIS2_PLACEMENT_3D('',#12040,#9467,#9468) ;
#7929=AXIS2_PLACEMENT_3D('',#12041,#9469,#9470) ;
#7930=AXIS2_PLACEMENT_3D('',#12043,#9471,#9472) ;
#7931=AXIS2_PLACEMENT_3D('',#12045,#9473,#9474) ;
#7932=AXIS2_PLACEMENT_3D('',#12046,#9475,#9476) ;
#7933=AXIS2_PLACEMENT_3D('',#12047,#9477,#9478) ;
#7934=AXIS2_PLACEMENT_3D('',#12049,#9479,#9480) ;
#7935=AXIS2_PLACEMENT_3D('',#12051,#9481,#9482) ;
#7936=AXIS2_PLACEMENT_3D('',#12052,#9483,#9484) ;
#7937=AXIS2_PLACEMENT_3D('',#12053,#9485,#9486) ;
#7938=AXIS2_PLACEMENT_3D('',#12055,#9488,#9489) ;
#7939=AXIS2_PLACEMENT_3D('',#12057,#9491,#9492) ;
#7940=AXIS2_PLACEMENT_3D('',#12059,#9494,#9495) ;
#7941=AXIS2_PLACEMENT_3D('',#12061,#9497,#9498) ;
#7942=AXIS2_PLACEMENT_3D('',#12066,#9500,#9501) ;
#7943=AXIS2_PLACEMENT_3D('',#12069,#9503,#9504) ;
#7944=AXIS2_PLACEMENT_3D('',#12070,#9505,#9506) ;
#7945=AXIS2_PLACEMENT_3D('',#12076,#9510,#9511) ;
#7946=AXIS2_PLACEMENT_3D('',#12078,#9512,#9513) ;
#7947=AXIS2_PLACEMENT_3D('',#12081,#9515,#9516) ;
#7948=AXIS2_PLACEMENT_3D('',#12082,#9517,#9518) ;
#7949=AXIS2_PLACEMENT_3D('',#12085,#9521,#9522) ;
#7950=AXIS2_PLACEMENT_3D('',#12090,#9524,#9525) ;
#7951=AXIS2_PLACEMENT_3D('',#12093,#9527,#9528) ;
#7952=AXIS2_PLACEMENT_3D('',#12094,#9529,#9530) ;
#7953=AXIS2_PLACEMENT_3D('',#12100,#9534,#9535) ;
#7954=AXIS2_PLACEMENT_3D('',#12102,#9536,#9537) ;
#7955=AXIS2_PLACEMENT_3D('',#12105,#9539,#9540) ;
#7956=AXIS2_PLACEMENT_3D('',#12106,#9541,#9542) ;
#7957=AXIS2_PLACEMENT_3D('',#12109,#9545,#9546) ;
#7958=AXIS2_PLACEMENT_3D('',#12114,#9548,#9549) ;
#7959=AXIS2_PLACEMENT_3D('',#12117,#9551,#9552) ;
#7960=AXIS2_PLACEMENT_3D('',#12118,#9553,#9554) ;
#7961=AXIS2_PLACEMENT_3D('',#12124,#9558,#9559) ;
#7962=AXIS2_PLACEMENT_3D('',#12126,#9560,#9561) ;
#7963=AXIS2_PLACEMENT_3D('',#12129,#9563,#9564) ;
#7964=AXIS2_PLACEMENT_3D('',#12130,#9565,#9566) ;
#7965=AXIS2_PLACEMENT_3D('',#12133,#9569,#9570) ;
#7966=AXIS2_PLACEMENT_3D('',#12142,#9575,#9576) ;
#7967=AXIS2_PLACEMENT_3D('',#12146,#9578,#9579) ;
#7968=AXIS2_PLACEMENT_3D('',#12147,#9580,#9581) ;
#7969=AXIS2_PLACEMENT_3D('',#12148,#9582,#9583) ;
#7970=AXIS2_PLACEMENT_3D('',#12154,#9587,#9588) ;
#7971=AXIS2_PLACEMENT_3D('',#12155,#9589,#9590) ;
#7972=AXIS2_PLACEMENT_3D('',#12156,#9591,#9592) ;
#7973=AXIS2_PLACEMENT_3D('',#12157,#9593,#9594) ;
#7974=AXIS2_PLACEMENT_3D('',#12166,#9599,#9600) ;
#7975=AXIS2_PLACEMENT_3D('',#12168,#9601,#9602) ;
#7976=AXIS2_PLACEMENT_3D('',#12171,#9604,#9605) ;
#7977=AXIS2_PLACEMENT_3D('',#12172,#9606,#9607) ;
#7978=AXIS2_PLACEMENT_3D('',#12178,#9611,#9612) ;
#7979=AXIS2_PLACEMENT_3D('',#12179,#9613,#9614) ;
#7980=AXIS2_PLACEMENT_3D('',#12180,#9615,#9616) ;
#7981=AXIS2_PLACEMENT_3D('',#12181,#9617,#9618) ;
#7982=AXIS2_PLACEMENT_3D('',#12190,#9623,#9624) ;
#7983=AXIS2_PLACEMENT_3D('',#12192,#9625,#9626) ;
#7984=AXIS2_PLACEMENT_3D('',#12195,#9628,#9629) ;
#7985=AXIS2_PLACEMENT_3D('',#12196,#9630,#9631) ;
#7986=AXIS2_PLACEMENT_3D('',#12202,#9635,#9636) ;
#7987=AXIS2_PLACEMENT_3D('',#12203,#9637,#9638) ;
#7988=AXIS2_PLACEMENT_3D('',#12204,#9639,#9640) ;
#7989=AXIS2_PLACEMENT_3D('',#12205,#9641,#9642) ;
#7990=AXIS2_PLACEMENT_3D('',#12214,#9647,#9648) ;
#7991=AXIS2_PLACEMENT_3D('',#12218,#9650,#9651) ;
#7992=AXIS2_PLACEMENT_3D('',#12219,#9652,#9653) ;
#7993=AXIS2_PLACEMENT_3D('',#12220,#9654,#9655) ;
#7994=AXIS2_PLACEMENT_3D('',#12226,#9659,#9660) ;
#7995=AXIS2_PLACEMENT_3D('',#12227,#9661,#9662) ;
#7996=AXIS2_PLACEMENT_3D('',#12228,#9663,#9664) ;
#7997=AXIS2_PLACEMENT_3D('',#12229,#9665,#9666) ;
#7998=AXIS2_PLACEMENT_3D('',#12238,#9671,#9672) ;
#7999=AXIS2_PLACEMENT_3D('',#12240,#9673,#9674) ;
#8000=AXIS2_PLACEMENT_3D('',#12243,#9676,#9677) ;
#8001=AXIS2_PLACEMENT_3D('',#12244,#9678,#9679) ;
#8002=AXIS2_PLACEMENT_3D('',#12250,#9683,#9684) ;
#8003=AXIS2_PLACEMENT_3D('',#12251,#9685,#9686) ;
#8004=AXIS2_PLACEMENT_3D('',#12252,#9687,#9688) ;
#8005=AXIS2_PLACEMENT_3D('',#12253,#9689,#9690) ;
#8006=AXIS2_PLACEMENT_3D('',#12254,#9691,#9692) ;
#8007=AXIS2_PLACEMENT_3D('',#12255,#9693,#9694) ;
#8008=AXIS2_PLACEMENT_3D('',#12256,#9695,#9696) ;
#8009=AXIS2_PLACEMENT_3D('',#12257,#9697,#9698) ;
#8010=AXIS2_PLACEMENT_3D('',#12258,#9699,#9700) ;
#8011=AXIS2_PLACEMENT_3D('',#12259,#9701,#9702) ;
#8012=AXIS2_PLACEMENT_3D('',#12262,#9703,#9704) ;
#8013=AXIS2_PLACEMENT_3D('',#12298,#9705,#9706) ;
#8014=AXIS2_PLACEMENT_3D('',#12300,#9708,#9709) ;
#8015=AXIS2_PLACEMENT_3D('',#12302,#9710,#9711) ;
#8016=AXIS2_PLACEMENT_3D('',#12303,#9712,#9713) ;
#8017=AXIS2_PLACEMENT_3D('',#12305,#9714,#9715) ;
#8018=AXIS2_PLACEMENT_3D('',#12306,#9716,#9717) ;
#8019=AXIS2_PLACEMENT_3D('',#12309,#9718,#9719) ;
#8020=AXIS2_PLACEMENT_3D('',#12311,#9720,#9721) ;
#8021=AXIS2_PLACEMENT_3D('',#12312,#9722,#9723) ;
#8022=AXIS2_PLACEMENT_3D('',#12314,#9724,#9725) ;
#8023=AXIS2_PLACEMENT_3D('',#12316,#9726,#9727) ;
#8024=AXIS2_PLACEMENT_3D('',#12318,#9728,#9729) ;
#8025=AXIS2_PLACEMENT_3D('',#12320,#9730,#9731) ;
#8026=AXIS2_PLACEMENT_3D('',#12321,#9732,#9733) ;
#8027=AXIS2_PLACEMENT_3D('',#12322,#9734,#9735) ;
#8028=AXIS2_PLACEMENT_3D('',#12323,#9736,#9737) ;
#8029=AXIS2_PLACEMENT_3D('',#12392,#9738,#9739) ;
#8030=AXIS2_PLACEMENT_3D('',#12394,#9740,#9741) ;
#8031=AXIS2_PLACEMENT_3D('',#12396,#9742,#9743) ;
#8032=AXIS2_PLACEMENT_3D('',#12397,#9744,#9745) ;
#8033=AXIS2_PLACEMENT_3D('',#12399,#9747,#9748) ;
#8034=AXIS2_PLACEMENT_3D('',#12401,#9750,#9751) ;
#8035=AXIS2_PLACEMENT_3D('',#12403,#9752,#9753) ;
#8036=AXIS2_PLACEMENT_3D('',#12405,#9754,#9755) ;
#8037=AXIS2_PLACEMENT_3D('',#12406,#9756,#9757) ;
#8038=AXIS2_PLACEMENT_3D('',#12408,#9759,#9760) ;
#9386=DIRECTION('axis',(0.,0.,1.)) ;
#9387=DIRECTION('refdir',(1.,0.,0.)) ;
#9388=DIRECTION('center_axis',(0.,0.,-1.)) ;
#9389=DIRECTION('ref_axis',(1.,0.,0.)) ;
#9390=DIRECTION('center_axis',(0.,0.,-1.)) ;
#9391=DIRECTION('ref_axis',(1.,0.,0.)) ;
#9392=DIRECTION('center_axis',(0.,0.,-1.)) ;
#9393=DIRECTION('ref_axis',(1.,0.,0.)) ;
#9394=DIRECTION('center_axis',(0.,0.,-1.)) ;
#9395=DIRECTION('ref_axis',(0.877582561890372,-0.479425538604204,0.)) ;
#9396=DIRECTION('',(0.,0.,-1.)) ;
#9397=DIRECTION('center_axis',(0.,0.,-1.)) ;
#9398=DIRECTION('ref_axis',(1.,0.,0.)) ;
#9399=DIRECTION('center_axis',(0.,0.,-1.)) ;
#9400=DIRECTION('ref_axis',(1.,0.,0.)) ;
#9401=DIRECTION('center_axis',(0.,0.,-1.)) ;
#9402=DIRECTION('ref_axis',(1.,0.,0.)) ;
#9403=DIRECTION('center_axis',(0.,0.,-1.)) ;
#9404=DIRECTION('ref_axis',(1.,0.,0.)) ;
#9405=DIRECTION('center_axis',(0.,0.,-1.)) ;
#9406=DIRECTION('ref_axis',(0.17323572618106,-0.984880390288344,0.)) ;
#9407=DIRECTION('center_axis',(0.,0.,-1.)) ;
#9408=DIRECTION('ref_axis',(1.,0.,0.)) ;
#9409=DIRECTION('',(0.,0.,-1.)) ;
#9410=DIRECTION('center_axis',(0.,0.,-1.)) ;
#9411=DIRECTION('ref_axis',(1.,0.,0.)) ;
#9412=DIRECTION('',(0.,0.,-1.)) ;
#9413=DIRECTION('',(0.,0.,-1.)) ;
#9414=DIRECTION('center_axis',(0.,0.,-1.)) ;
#9415=DIRECTION('ref_axis',(1.,0.,0.)) ;
#9416=DIRECTION('',(0.,0.,-1.)) ;
#9417=DIRECTION('center_axis',(0.,0.,-1.)) ;
#9418=DIRECTION('ref_axis',(3.96508223080413E-16,1.,0.)) ;
#9419=DIRECTION('center_axis',(0.,0.,-1.)) ;
#9420=DIRECTION('ref_axis',(1.,0.,0.)) ;
#9421=DIRECTION('center_axis',(0.,0.,-1.)) ;
#9422=DIRECTION('ref_axis',(-0.479425538604204,-0.877582561890372,0.)) ;
#9423=DIRECTION('center_axis',(0.,0.,-1.)) ;
#9424=DIRECTION('ref_axis',(1.,0.,0.)) ;
#9425=DIRECTION('center_axis',(0.,0.,-1.)) ;
#9426=DIRECTION('ref_axis',(1.,0.,0.)) ;
#9427=DIRECTION('center_axis',(0.,0.,-1.)) ;
#9428=DIRECTION('ref_axis',(1.,0.,0.)) ;
#9429=DIRECTION('center_axis',(0.,0.,-1.)) ;
#9430=DIRECTION('ref_axis',(1.,0.,0.)) ;
#9431=DIRECTION('center_axis',(0.,0.,-1.)) ;
#9432=DIRECTION('ref_axis',(1.,0.,0.)) ;
#9433=DIRECTION('center_axis',(0.,0.,-1.)) ;
#9434=DIRECTION('ref_axis',(1.,0.,0.)) ;
#9435=DIRECTION('',(0.00775534185661509,0.0141960580462165,-0.999869154744077)) ;
#9436=DIRECTION('center_axis',(0.,0.,-1.)) ;
#9437=DIRECTION('ref_axis',(1.,0.,0.)) ;
#9438=DIRECTION('center_axis',(0.,0.,-1.)) ;
#9439=DIRECTION('ref_axis',(-2.92163953848725E-17,1.,0.)) ;
#9440=DIRECTION('center_axis',(0.,0.,-1.)) ;
#9441=DIRECTION('ref_axis',(1.,0.,0.)) ;
#9442=DIRECTION('center_axis',(0.,0.,-1.)) ;
#9443=DIRECTION('ref_axis',(1.,0.,0.)) ;
#9444=DIRECTION('center_axis',(0.,0.,-1.)) ;
#9445=DIRECTION('ref_axis',(1.,0.,0.)) ;
#9446=DIRECTION('center_axis',(0.,0.,-1.)) ;
#9447=DIRECTION('ref_axis',(1.,0.,0.)) ;
#9448=DIRECTION('center_axis',(0.,0.,-1.)) ;
#9449=DIRECTION('ref_axis',(-0.479425538604204,-0.877582561890372,0.)) ;
#9450=DIRECTION('',(-0.00775534185661509,-0.0141960580462165,0.999869154744077)) ;
#9451=DIRECTION('center_axis',(0.,0.,-1.)) ;
#9452=DIRECTION('ref_axis',(1.,0.,0.)) ;
#9453=DIRECTION('center_axis',(0.,0.,-1.)) ;
#9454=DIRECTION('ref_axis',(-0.866025403784633,-0.499999999999664,0.)) ;
#9455=DIRECTION('',(0.,0.,-1.)) ;
#9456=DIRECTION('center_axis',(0.,0.,-1.)) ;
#9457=DIRECTION('ref_axis',(1.,0.,0.)) ;
#9458=DIRECTION('',(0.,0.,-1.)) ;
#9459=DIRECTION('center_axis',(0.,0.,-1.)) ;
#9460=DIRECTION('ref_axis',(1.,0.,0.)) ;
#9461=DIRECTION('center_axis',(0.,0.,-1.)) ;
#9462=DIRECTION('ref_axis',(0.866025403784633,-0.499999999999663,0.)) ;
#9463=DIRECTION('',(0.,0.,-1.)) ;
#9464=DIRECTION('center_axis',(0.,0.,-1.)) ;
#9465=DIRECTION('ref_axis',(1.,0.,0.)) ;
#9466=DIRECTION('',(0.,0.,-1.)) ;
#9467=DIRECTION('center_axis',(0.,0.,-1.)) ;
#9468=DIRECTION('ref_axis',(1.,0.,0.)) ;
#9469=DIRECTION('center_axis',(0.,0.,-1.)) ;
#9470=DIRECTION('ref_axis',(1.,0.,0.)) ;
#9471=DIRECTION('center_axis',(0.,0.,-1.)) ;
#9472=DIRECTION('ref_axis',(1.,0.,0.)) ;
#9473=DIRECTION('center_axis',(0.,0.,-1.)) ;
#9474=DIRECTION('ref_axis',(1.,0.,0.)) ;
#9475=DIRECTION('center_axis',(0.,0.,-1.)) ;
#9476=DIRECTION('ref_axis',(1.,0.,0.)) ;
#9477=DIRECTION('center_axis',(0.,0.,-1.)) ;
#9478=DIRECTION('ref_axis',(1.,0.,0.)) ;
#9479=DIRECTION('center_axis',(0.,0.,-1.)) ;
#9480=DIRECTION('ref_axis',(1.,0.,0.)) ;
#9481=DIRECTION('center_axis',(0.,0.,-1.)) ;
#9482=DIRECTION('ref_axis',(1.,0.,0.)) ;
#9483=DIRECTION('center_axis',(0.,0.,-1.)) ;
#9484=DIRECTION('ref_axis',(1.,0.,0.)) ;
#9485=DIRECTION('center_axis',(0.,0.,-1.)) ;
#9486=DIRECTION('ref_axis',(0.866025403786762,-0.499999999995976,0.)) ;
#9487=DIRECTION('',(0.,0.,-1.)) ;
#9488=DIRECTION('center_axis',(0.,0.,-1.)) ;
#9489=DIRECTION('ref_axis',(1.,0.,0.)) ;
#9490=DIRECTION('',(0.,0.,-1.)) ;
#9491=DIRECTION('center_axis',(0.,0.,-1.)) ;
#9492=DIRECTION('ref_axis',(-0.866025403786762,-0.499999999995976,0.)) ;
#9493=DIRECTION('',(0.,0.,-1.)) ;
#9494=DIRECTION('center_axis',(0.,0.,-1.)) ;
#9495=DIRECTION('ref_axis',(1.,0.,0.)) ;
#9496=DIRECTION('',(0.,0.,-1.)) ;
#9497=DIRECTION('center_axis',(0.,0.,1.)) ;
#9498=DIRECTION('ref_axis',(-0.120967741934967,0.992656438759733,0.)) ;
#9499=DIRECTION('',(0.,0.,1.)) ;
#9500=DIRECTION('center_axis',(0.,0.,1.)) ;
#9501=DIRECTION('ref_axis',(-1.,0.,0.)) ;
#9502=DIRECTION('',(0.,0.,1.)) ;
#9503=DIRECTION('center_axis',(0.,0.,1.)) ;
#9504=DIRECTION('ref_axis',(-1.,0.,0.)) ;
#9505=DIRECTION('center_axis',(1.,0.,0.)) ;
#9506=DIRECTION('ref_axis',(0.,-1.,0.)) ;
#9507=DIRECTION('',(0.,-1.,0.)) ;
#9508=DIRECTION('',(0.,0.,-1.)) ;
#9509=DIRECTION('',(0.,-1.,0.)) ;
#9510=DIRECTION('center_axis',(0.,0.,1.)) ;
#9511=DIRECTION('ref_axis',(-0.102040816326951,0.994780212812523,0.)) ;
#9512=DIRECTION('center_axis',(0.,0.,1.)) ;
#9513=DIRECTION('ref_axis',(-1.,0.,0.)) ;
#9514=DIRECTION('',(0.,0.,1.)) ;
#9515=DIRECTION('center_axis',(0.,0.,1.)) ;
#9516=DIRECTION('ref_axis',(-1.,0.,0.)) ;
#9517=DIRECTION('center_axis',(0.,1.,0.)) ;
#9518=DIRECTION('ref_axis',(1.,0.,0.)) ;
#9519=DIRECTION('',(1.,0.,0.)) ;
#9520=DIRECTION('',(1.,0.,0.)) ;
#9521=DIRECTION('center_axis',(0.,0.,1.)) ;
#9522=DIRECTION('ref_axis',(-0.202702702702927,0.979240325107646,0.)) ;
#9523=DIRECTION('',(0.,0.,1.)) ;
#9524=DIRECTION('center_axis',(0.,0.,1.)) ;
#9525=DIRECTION('ref_axis',(-1.,0.,0.)) ;
#9526=DIRECTION('',(0.,0.,1.)) ;
#9527=DIRECTION('center_axis',(0.,0.,1.)) ;
#9528=DIRECTION('ref_axis',(-1.,0.,0.)) ;
#9529=DIRECTION('center_axis',(1.,0.,0.)) ;
#9530=DIRECTION('ref_axis',(0.,-1.,0.)) ;
#9531=DIRECTION('',(0.,-1.,0.)) ;
#9532=DIRECTION('',(0.,0.,-1.)) ;
#9533=DIRECTION('',(0.,-1.,0.)) ;
#9534=DIRECTION('center_axis',(0.,0.,1.)) ;
#9535=DIRECTION('ref_axis',(-0.154639175257936,0.987971014491592,0.)) ;
#9536=DIRECTION('center_axis',(0.,0.,1.)) ;
#9537=DIRECTION('ref_axis',(-1.,0.,0.)) ;
#9538=DIRECTION('',(0.,0.,1.)) ;
#9539=DIRECTION('center_axis',(0.,0.,1.)) ;
#9540=DIRECTION('ref_axis',(-1.,0.,0.)) ;
#9541=DIRECTION('center_axis',(0.,1.,0.)) ;
#9542=DIRECTION('ref_axis',(1.,0.,0.)) ;
#9543=DIRECTION('',(1.,0.,0.)) ;
#9544=DIRECTION('',(1.,0.,0.)) ;
#9545=DIRECTION('center_axis',(0.,0.,1.)) ;
#9546=DIRECTION('ref_axis',(-0.120967741934967,0.992656438759733,0.)) ;
#9547=DIRECTION('',(0.,0.,1.)) ;
#9548=DIRECTION('center_axis',(0.,0.,1.)) ;
#9549=DIRECTION('ref_axis',(-1.,0.,0.)) ;
#9550=DIRECTION('',(0.,0.,1.)) ;
#9551=DIRECTION('center_axis',(0.,0.,1.)) ;
#9552=DIRECTION('ref_axis',(-1.,0.,0.)) ;
#9553=DIRECTION('center_axis',(0.,1.,0.)) ;
#9554=DIRECTION('ref_axis',(1.,0.,0.)) ;
#9555=DIRECTION('',(0.,0.,-1.)) ;
#9556=DIRECTION('',(1.,0.,0.)) ;
#9557=DIRECTION('',(1.,0.,0.)) ;
#9558=DIRECTION('center_axis',(0.,0.,1.)) ;
#9559=DIRECTION('ref_axis',(-0.102040816326951,0.994780212812523,0.)) ;
#9560=DIRECTION('center_axis',(0.,0.,1.)) ;
#9561=DIRECTION('ref_axis',(-1.,0.,0.)) ;
#9562=DIRECTION('',(0.,0.,1.)) ;
#9563=DIRECTION('center_axis',(0.,0.,1.)) ;
#9564=DIRECTION('ref_axis',(-1.,0.,0.)) ;
#9565=DIRECTION('center_axis',(1.,0.,0.)) ;
#9566=DIRECTION('ref_axis',(0.,-1.,0.)) ;
#9567=DIRECTION('',(0.,-1.,0.)) ;
#9568=DIRECTION('',(0.,-1.,0.)) ;
#9569=DIRECTION('center_axis',(0.,1.,0.)) ;
#9570=DIRECTION('ref_axis',(1.,0.,0.)) ;
#9571=DIRECTION('',(0.,0.,-1.)) ;
#9572=DIRECTION('',(1.,0.,0.)) ;
#9573=DIRECTION('',(0.,0.,-1.)) ;
#9574=DIRECTION('',(1.,0.,0.)) ;
#9575=DIRECTION('center_axis',(0.,0.,1.)) ;
#9576=DIRECTION('ref_axis',(0.992656438759733,0.120967741934967,0.)) ;
#9577=DIRECTION('',(0.,0.,1.)) ;
#9578=DIRECTION('center_axis',(0.,0.,1.)) ;
#9579=DIRECTION('ref_axis',(-1.,0.,0.)) ;
#9580=DIRECTION('center_axis',(0.,0.,1.)) ;
#9581=DIRECTION('ref_axis',(-1.,0.,0.)) ;
#9582=DIRECTION('center_axis',(1.,0.,0.)) ;
#9583=DIRECTION('ref_axis',(0.,-1.,0.)) ;
#9584=DIRECTION('',(0.,0.,-1.)) ;
#9585=DIRECTION('',(0.,-1.,0.)) ;
#9586=DIRECTION('',(0.,-1.,0.)) ;
#9587=DIRECTION('center_axis',(0.,0.,1.)) ;
#9588=DIRECTION('ref_axis',(0.994780212812523,0.102040816326951,0.)) ;
#9589=DIRECTION('center_axis',(0.,0.,1.)) ;
#9590=DIRECTION('ref_axis',(-1.,0.,0.)) ;
#9591=DIRECTION('center_axis',(0.,0.,1.)) ;
#9592=DIRECTION('ref_axis',(-1.,0.,0.)) ;
#9593=DIRECTION('center_axis',(0.,1.,0.)) ;
#9594=DIRECTION('ref_axis',(1.,0.,0.)) ;
#9595=DIRECTION('',(1.,0.,0.)) ;
#9596=DIRECTION('',(0.,0.,-1.)) ;
#9597=DIRECTION('',(1.,0.,0.)) ;
#9598=DIRECTION('',(0.,0.,-1.)) ;
#9599=DIRECTION('center_axis',(0.,0.,1.)) ;
#9600=DIRECTION('ref_axis',(-0.154639175257936,0.987971014491592,0.)) ;
#9601=DIRECTION('center_axis',(0.,0.,1.)) ;
#9602=DIRECTION('ref_axis',(-1.,0.,0.)) ;
#9603=DIRECTION('',(0.,0.,1.)) ;
#9604=DIRECTION('center_axis',(0.,0.,1.)) ;
#9605=DIRECTION('ref_axis',(-1.,0.,0.)) ;
#9606=DIRECTION('center_axis',(1.,0.,0.)) ;
#9607=DIRECTION('ref_axis',(0.,-1.,0.)) ;
#9608=DIRECTION('',(0.,0.,-1.)) ;
#9609=DIRECTION('',(0.,-1.,0.)) ;
#9610=DIRECTION('',(0.,-1.,0.)) ;
#9611=DIRECTION('center_axis',(0.,0.,1.)) ;
#9612=DIRECTION('ref_axis',(-0.202702702702927,0.979240325107646,0.)) ;
#9613=DIRECTION('center_axis',(0.,0.,1.)) ;
#9614=DIRECTION('ref_axis',(-1.,0.,0.)) ;
#9615=DIRECTION('center_axis',(0.,0.,1.)) ;
#9616=DIRECTION('ref_axis',(-1.,0.,0.)) ;
#9617=DIRECTION('center_axis',(1.,0.,0.)) ;
#9618=DIRECTION('ref_axis',(0.,-1.,0.)) ;
#9619=DIRECTION('',(0.,0.,-1.)) ;
#9620=DIRECTION('',(0.,-1.,0.)) ;
#9621=DIRECTION('',(0.,0.,-1.)) ;
#9622=DIRECTION('',(0.,-1.,0.)) ;
#9623=DIRECTION('center_axis',(0.,0.,1.)) ;
#9624=DIRECTION('ref_axis',(0.987971014491592,0.154639175257936,0.)) ;
#9625=DIRECTION('center_axis',(0.,0.,1.)) ;
#9626=DIRECTION('ref_axis',(-1.,0.,0.)) ;
#9627=DIRECTION('',(0.,0.,1.)) ;
#9628=DIRECTION('center_axis',(0.,0.,1.)) ;
#9629=DIRECTION('ref_axis',(-1.,0.,0.)) ;
#9630=DIRECTION('center_axis',(0.,1.,0.)) ;
#9631=DIRECTION('ref_axis',(1.,0.,0.)) ;
#9632=DIRECTION('',(0.,0.,-1.)) ;
#9633=DIRECTION('',(1.,0.,0.)) ;
#9634=DIRECTION('',(1.,0.,0.)) ;
#9635=DIRECTION('center_axis',(0.,0.,1.)) ;
#9636=DIRECTION('ref_axis',(0.979240325107646,0.202702702702927,0.)) ;
#9637=DIRECTION('center_axis',(0.,0.,1.)) ;
#9638=DIRECTION('ref_axis',(-1.,0.,0.)) ;
#9639=DIRECTION('center_axis',(0.,0.,1.)) ;
#9640=DIRECTION('ref_axis',(-1.,0.,0.)) ;
#9641=DIRECTION('center_axis',(1.,0.,0.)) ;
#9642=DIRECTION('ref_axis',(0.,-1.,0.)) ;
#9643=DIRECTION('',(0.,-1.,0.)) ;
#9644=DIRECTION('',(0.,0.,-1.)) ;
#9645=DIRECTION('',(0.,-1.,0.)) ;
#9646=DIRECTION('',(0.,0.,-1.)) ;
#9647=DIRECTION('center_axis',(0.,0.,1.)) ;
#9648=DIRECTION('ref_axis',(-0.202702702702927,0.979240325107646,0.)) ;
#9649=DIRECTION('',(0.,0.,1.)) ;
#9650=DIRECTION('center_axis',(0.,0.,1.)) ;
#9651=DIRECTION('ref_axis',(-1.,0.,0.)) ;
#9652=DIRECTION('center_axis',(0.,0.,1.)) ;
#9653=DIRECTION('ref_axis',(-1.,0.,0.)) ;
#9654=DIRECTION('center_axis',(0.,1.,0.)) ;
#9655=DIRECTION('ref_axis',(1.,0.,0.)) ;
#9656=DIRECTION('',(0.,0.,-1.)) ;
#9657=DIRECTION('',(1.,0.,0.)) ;
#9658=DIRECTION('',(1.,0.,0.)) ;
#9659=DIRECTION('center_axis',(0.,0.,1.)) ;
#9660=DIRECTION('ref_axis',(-0.154639175257936,0.987971014491592,0.)) ;
#9661=DIRECTION('center_axis',(0.,0.,1.)) ;
#9662=DIRECTION('ref_axis',(-1.,0.,0.)) ;
#9663=DIRECTION('center_axis',(0.,0.,1.)) ;
#9664=DIRECTION('ref_axis',(-1.,0.,0.)) ;
#9665=DIRECTION('center_axis',(0.,1.,0.)) ;
#9666=DIRECTION('ref_axis',(1.,0.,0.)) ;
#9667=DIRECTION('',(1.,0.,0.)) ;
#9668=DIRECTION('',(0.,0.,-1.)) ;
#9669=DIRECTION('',(1.,0.,0.)) ;
#9670=DIRECTION('',(0.,0.,-1.)) ;
#9671=DIRECTION('center_axis',(0.,0.,1.)) ;
#9672=DIRECTION('ref_axis',(-0.102040816326951,0.994780212812523,0.)) ;
#9673=DIRECTION('center_axis',(0.,0.,1.)) ;
#9674=DIRECTION('ref_axis',(-1.,0.,0.)) ;
#9675=DIRECTION('',(0.,0.,1.)) ;
#9676=DIRECTION('center_axis',(0.,0.,1.)) ;
#9677=DIRECTION('ref_axis',(-1.,0.,0.)) ;
#9678=DIRECTION('center_axis',(1.,0.,0.)) ;
#9679=DIRECTION('ref_axis',(0.,-1.,0.)) ;
#9680=DIRECTION('',(0.,0.,-1.)) ;
#9681=DIRECTION('',(0.,-1.,0.)) ;
#9682=DIRECTION('',(0.,-1.,0.)) ;
#9683=DIRECTION('center_axis',(0.,0.,1.)) ;
#9684=DIRECTION('ref_axis',(-0.120967741934967,0.992656438759733,0.)) ;
#9685=DIRECTION('center_axis',(0.,0.,1.)) ;
#9686=DIRECTION('ref_axis',(-1.,0.,0.)) ;
#9687=DIRECTION('center_axis',(0.,0.,1.)) ;
#9688=DIRECTION('ref_axis',(-1.,0.,0.)) ;
#9689=DIRECTION('center_axis',(0.,0.,-1.)) ;
#9690=DIRECTION('ref_axis',(-0.920196061075712,0.391457799999878,0.)) ;
#9691=DIRECTION('center_axis',(0.,0.,-1.)) ;
#9692=DIRECTION('ref_axis',(1.,0.,0.)) ;
#9693=DIRECTION('center_axis',(0.,0.,-1.)) ;
#9694=DIRECTION('ref_axis',(0.766313574588188,0.642466734860158,0.)) ;
#9695=DIRECTION('center_axis',(0.,0.,-1.)) ;
#9696=DIRECTION('ref_axis',(1.,0.,0.)) ;
#9697=DIRECTION('center_axis',(0.,0.,-1.)) ;
#9698=DIRECTION('ref_axis',(1.,0.,0.)) ;
#9699=DIRECTION('center_axis',(0.,0.,-1.)) ;
#9700=DIRECTION('ref_axis',(1.,0.,0.)) ;
#9701=DIRECTION('center_axis',(0.,0.,-1.)) ;
#9702=DIRECTION('ref_axis',(0.877582561890373,-0.479425538604203,0.)) ;
#9703=DIRECTION('center_axis',(0.,0.,-1.)) ;
#9704=DIRECTION('ref_axis',(1.,0.,0.)) ;
#9705=DIRECTION('center_axis',(0.,0.,-1.)) ;
#9706=DIRECTION('ref_axis',(1.,0.,0.)) ;
#9707=DIRECTION('',(0.,0.,-1.)) ;
#9708=DIRECTION('center_axis',(0.,0.,-1.)) ;
#9709=DIRECTION('ref_axis',(1.,0.,0.)) ;
#9710=DIRECTION('center_axis',(0.,0.,-1.)) ;
#9711=DIRECTION('ref_axis',(1.,0.,0.)) ;
#9712=DIRECTION('center_axis',(0.,0.,-1.)) ;
#9713=DIRECTION('ref_axis',(1.,0.,0.)) ;
#9714=DIRECTION('center_axis',(0.,0.,-1.)) ;
#9715=DIRECTION('ref_axis',(1.,0.,0.)) ;
#9716=DIRECTION('center_axis',(0.,0.,-1.)) ;
#9717=DIRECTION('ref_axis',(1.,0.,0.)) ;
#9718=DIRECTION('center_axis',(0.,0.,-1.)) ;
#9719=DIRECTION('ref_axis',(1.,0.,0.)) ;
#9720=DIRECTION('center_axis',(0.,0.,-1.)) ;
#9721=DIRECTION('ref_axis',(1.,0.,0.)) ;
#9722=DIRECTION('center_axis',(0.,0.,-1.)) ;
#9723=DIRECTION('ref_axis',(1.,0.,0.)) ;
#9724=DIRECTION('center_axis',(0.,0.,-1.)) ;
#9725=DIRECTION('ref_axis',(1.,0.,0.)) ;
#9726=DIRECTION('center_axis',(0.,0.,-1.)) ;
#9727=DIRECTION('ref_axis',(1.,0.,0.)) ;
#9728=DIRECTION('center_axis',(0.,0.,-1.)) ;
#9729=DIRECTION('ref_axis',(1.,0.,0.)) ;
#9730=DIRECTION('center_axis',(0.,0.,-1.)) ;
#9731=DIRECTION('ref_axis',(1.,0.,0.)) ;
#9732=DIRECTION('center_axis',(0.,0.,-1.)) ;
#9733=DIRECTION('ref_axis',(1.,0.,0.)) ;
#9734=DIRECTION('center_axis',(0.,0.,-1.)) ;
#9735=DIRECTION('ref_axis',(-0.479425538604204,-0.877582561890372,0.)) ;
#9736=DIRECTION('center_axis',(0.877582561890372,-0.479425538604204,0.)) ;
#9737=DIRECTION('ref_axis',(0.479425538604204,0.877582561890372,0.)) ;
#9738=DIRECTION('center_axis',(0.,0.,-1.)) ;
#9739=DIRECTION('ref_axis',(1.,0.,0.)) ;
#9740=DIRECTION('center_axis',(0.,0.,-1.)) ;
#9741=DIRECTION('ref_axis',(1.,0.,0.)) ;
#9742=DIRECTION('center_axis',(0.,0.,-1.)) ;
#9743=DIRECTION('ref_axis',(1.,0.,0.)) ;
#9744=DIRECTION('center_axis',(0.,0.,-1.)) ;
#9745=DIRECTION('ref_axis',(-0.0235965852909093,0.999721561817394,0.)) ;
#9746=DIRECTION('',(0.,0.,-1.)) ;
#9747=DIRECTION('center_axis',(0.,0.,-1.)) ;
#9748=DIRECTION('ref_axis',(-0.0235965852909093,0.999721561817394,0.)) ;
#9749=DIRECTION('',(0.,0.,-1.)) ;
#9750=DIRECTION('center_axis',(0.,0.,-1.)) ;
#9751=DIRECTION('ref_axis',(1.,0.,0.)) ;
#9752=DIRECTION('center_axis',(0.,0.,-1.)) ;
#9753=DIRECTION('ref_axis',(1.,0.,0.)) ;
#9754=DIRECTION('center_axis',(0.,0.,-1.)) ;
#9755=DIRECTION('ref_axis',(1.,0.,0.)) ;
#9756=DIRECTION('center_axis',(0.,0.,-1.)) ;
#9757=DIRECTION('ref_axis',(-0.853985976599423,-0.520296023213257,0.)) ;
#9758=DIRECTION('',(0.,0.,-1.)) ;
#9759=DIRECTION('center_axis',(0.,0.,-1.)) ;
#9760=DIRECTION('ref_axis',(-0.853985976599423,-0.520296023213258,0.)) ;
#9761=DIRECTION('',(0.,0.,-1.)) ;
#11967=CARTESIAN_POINT('',(0.,0.,0.)) ;
#11968=CARTESIAN_POINT('Origin',(1.55,-25.,142.2)) ;
#11969=CARTESIAN_POINT('',(-2.45723117329,-23.6576084919,142.2)) ;
#11970=CARTESIAN_POINT('Origin',(0.,-25.,142.2)) ;
#11971=CARTESIAN_POINT('',(-1.36025297093008,-24.2568904151635,142.2)) ;
#11972=CARTESIAN_POINT('Origin',(0.,-25.,142.2)) ;
#11973=CARTESIAN_POINT('Origin',(0.,-25.,144.1)) ;
#11974=CARTESIAN_POINT('',(-1.36025297093008,-24.2568904151635,139.1)) ;
#11975=CARTESIAN_POINT('',(-1.36025297093008,-24.2568904151635,144.1)) ;
#11976=CARTESIAN_POINT('Origin',(0.,-25.,139.1)) ;
#11977=CARTESIAN_POINT('Origin',(0.,0.,139.1)) ;
#11978=CARTESIAN_POINT('',(3.2175930105,-26.3773507973,139.1)) ;
#11979=CARTESIAN_POINT('',(-3.2175930105,-26.3773507973,139.1)) ;
#11980=CARTESIAN_POINT('Origin',(0.,0.,139.1)) ;
#11981=CARTESIAN_POINT('Origin',(0.,-25.,139.1)) ;
#11982=CARTESIAN_POINT('Origin',(0.,0.,140.2)) ;
#11983=CARTESIAN_POINT('',(4.60337082176,-26.1711007973,141.3)) ;
#11984=CARTESIAN_POINT('',(-4.60337082213,-26.1711007972,141.3)) ;
#11985=CARTESIAN_POINT('Origin',(0.,0.,141.3)) ;
#11986=CARTESIAN_POINT('',(-4.60337082176,-26.1711007973,140.3)) ;
#11987=CARTESIAN_POINT('',(-4.60337082176,-26.1711007973,140.2)) ;
#11988=CARTESIAN_POINT('',(-3.2175930105,-26.3773507973,140.3)) ;
#11989=CARTESIAN_POINT('Origin',(0.,0.,140.3)) ;
#11990=CARTESIAN_POINT('',(-3.2175930105,-26.3773507973,140.2)) ;
#11991=CARTESIAN_POINT('',(3.2175930105,-26.3773507973,140.3)) ;
#11992=CARTESIAN_POINT('',(3.2175930105,-26.3773507973,140.2)) ;
#11993=CARTESIAN_POINT('',(4.60337082176,-26.1711007973,140.3)) ;
#11994=CARTESIAN_POINT('Origin',(0.,0.,140.3)) ;
#11995=CARTESIAN_POINT('',(4.60337082176,-26.1711007973,140.2)) ;
#11996=CARTESIAN_POINT('Origin',(0.,-25.,140.2)) ;
#11997=CARTESIAN_POINT('Origin',(0.,-25.,140.3)) ;
#11998=CARTESIAN_POINT('Origin',(0.,0.,141.3)) ;
#11999=CARTESIAN_POINT('',(-20.3631527246,17.0721864733,141.3)) ;
#12000=CARTESIAN_POINT('',(12.7397135929703,23.3198893100652,141.3)) ;
#12001=CARTESIAN_POINT('Origin',(0.,0.,141.3)) ;
#12002=CARTESIAN_POINT('',(-24.9665235463,9.09891432396,141.3)) ;
#12003=CARTESIAN_POINT('Origin',(0.,0.,141.3)) ;
#12004=CARTESIAN_POINT('Origin',(0.,0.,141.3)) ;
#12005=CARTESIAN_POINT('',(24.9665235463,9.09891432396,141.3)) ;
#12006=CARTESIAN_POINT('Origin',(0.,0.,141.3)) ;
#12007=CARTESIAN_POINT('',(20.3631527246,17.0721864733,141.3)) ;
#12008=CARTESIAN_POINT('Origin',(0.,0.,141.3)) ;
#12009=CARTESIAN_POINT('Origin',(0.,0.,141.3)) ;
#12010=CARTESIAN_POINT('',(12.920436705,23.6507007476,118.)) ;
#12011=CARTESIAN_POINT('',(12.7397135929703,23.3198893100652,141.3)) ;
#12012=CARTESIAN_POINT('Origin',(0.,0.,118.)) ;
#12013=CARTESIAN_POINT('Origin',(0.,-25.,140.8)) ;
#12014=CARTESIAN_POINT('Origin',(0.,-25.,141.3)) ;
#12015=CARTESIAN_POINT('Origin',(0.,-25.,140.3)) ;
#12016=CARTESIAN_POINT('Origin',(0.,-26.9498298789,118.)) ;
#12017=CARTESIAN_POINT('',(13.5437714656,24.7917073734,118.)) ;
#12018=CARTESIAN_POINT('Origin',(0.,0.,118.)) ;
#12019=CARTESIAN_POINT('Origin',(0.,0.,142.724264483)) ;
#12020=CARTESIAN_POINT('',(13.3520012501,24.4406743486,142.724264483)) ;
#12021=CARTESIAN_POINT('',(13.3520012501271,24.4406743486469,142.724264483)) ;
#12022=CARTESIAN_POINT('Origin',(0.,0.,142.724264483)) ;
#12023=CARTESIAN_POINT('Origin',(21.6506350946,12.5,140.2)) ;
#12024=CARTESIAN_POINT('',(21.2346593697,15.9751926848,140.3)) ;
#12025=CARTESIAN_POINT('',(21.2346593697,15.9751926848,139.1)) ;
#12026=CARTESIAN_POINT('',(21.2346593697,15.9751926848,140.2)) ;
#12027=CARTESIAN_POINT('',(24.4522523802,10.4021581125,139.1)) ;
#12028=CARTESIAN_POINT('Origin',(21.6506350946,12.5,139.1)) ;
#12029=CARTESIAN_POINT('',(24.4522523802,10.4021581125,140.3)) ;
#12030=CARTESIAN_POINT('',(24.4522523802,10.4021581125,140.2)) ;
#12031=CARTESIAN_POINT('Origin',(21.6506350946,12.5,140.3)) ;
#12032=CARTESIAN_POINT('Origin',(-21.6506350946,12.5,140.2)) ;
#12033=CARTESIAN_POINT('',(-24.4522523802,10.4021581125,140.3)) ;
#12034=CARTESIAN_POINT('',(-24.4522523802,10.4021581125,139.1)) ;
#12035=CARTESIAN_POINT('',(-24.4522523802,10.4021581125,140.2)) ;
#12036=CARTESIAN_POINT('',(-21.2346593697,15.9751926848,139.1)) ;
#12037=CARTESIAN_POINT('Origin',(-21.6506350946,12.5,139.1)) ;
#12038=CARTESIAN_POINT('',(-21.2346593697,15.9751926848,140.3)) ;
#12039=CARTESIAN_POINT('',(-21.2346593697,15.9751926848,140.2)) ;
#12040=CARTESIAN_POINT('Origin',(-21.6506350946,12.5,140.3)) ;
#12041=CARTESIAN_POINT('Origin',(0.,0.,140.3)) ;
#12042=CARTESIAN_POINT('',(-20.3631527246,17.0721864733,140.3)) ;
#12043=CARTESIAN_POINT('Origin',(3.5527136788E-15,0.,140.3)) ;
#12044=CARTESIAN_POINT('',(-24.9665235463,9.09891432396,140.3)) ;
#12045=CARTESIAN_POINT('Origin',(-21.6506350946,12.5,140.3)) ;
#12046=CARTESIAN_POINT('Origin',(3.5527136788E-15,0.,140.3)) ;
#12047=CARTESIAN_POINT('Origin',(0.,0.,140.3)) ;
#12048=CARTESIAN_POINT('',(24.9665235463,9.09891432396,140.3)) ;
#12049=CARTESIAN_POINT('Origin',(0.,0.,140.3)) ;
#12050=CARTESIAN_POINT('',(20.3631527246,17.0721864733,140.3)) ;
#12051=CARTESIAN_POINT('Origin',(21.6506350946,12.5,140.3)) ;
#12052=CARTESIAN_POINT('Origin',(0.,0.,140.3)) ;
#12053=CARTESIAN_POINT('Origin',(-21.6506350946,12.5,140.8)) ;
#12054=CARTESIAN_POINT('',(-20.3631527246,17.0721864733,140.8)) ;
#12055=CARTESIAN_POINT('Origin',(-21.6506350946,12.5,141.3)) ;
#12056=CARTESIAN_POINT('',(-24.9665235463,9.09891432396,140.8)) ;
#12057=CARTESIAN_POINT('Origin',(21.6506350946,12.5,140.8)) ;
#12058=CARTESIAN_POINT('',(24.9665235463,9.09891432396,140.8)) ;
#12059=CARTESIAN_POINT('Origin',(21.6506350946,12.5,141.3)) ;
#12060=CARTESIAN_POINT('',(20.3631527246,17.0721864733,140.8)) ;
#12061=CARTESIAN_POINT('Origin',(0.,0.,130.439999998)) ;
#12062=CARTESIAN_POINT('',(-1.5,-12.3089398406,144.2)) ;
#12063=CARTESIAN_POINT('',(-1.5,-12.3089398406,141.3)) ;
#12064=CARTESIAN_POINT('',(-1.5,-12.3089398406,130.439999998)) ;
#12065=CARTESIAN_POINT('',(-12.3089398406,-1.5,144.2)) ;
#12066=CARTESIAN_POINT('Origin',(0.,0.,144.2)) ;
#12067=CARTESIAN_POINT('',(-12.3089398406,-1.5,141.3)) ;
#12068=CARTESIAN_POINT('',(-12.3089398406,-1.5,130.439999998)) ;
#12069=CARTESIAN_POINT('Origin',(0.,0.,141.3)) ;
#12070=CARTESIAN_POINT('Origin',(-1.5,-12.3089398406,144.2)) ;
#12071=CARTESIAN_POINT('',(-1.5,-14.6232691283,141.3)) ;
#12072=CARTESIAN_POINT('',(-1.5,-13.4661044845,141.3)) ;
#12073=CARTESIAN_POINT('',(-1.5,-14.6232691283,144.2)) ;
#12074=CARTESIAN_POINT('',(-1.5,-14.6232691283,142.75)) ;
#12075=CARTESIAN_POINT('',(-1.5,-13.4661044845,144.2)) ;
#12076=CARTESIAN_POINT('Origin',(0.,0.,130.439999998)) ;
#12077=CARTESIAN_POINT('',(-14.6232691283,-1.5,141.3)) ;
#12078=CARTESIAN_POINT('Origin',(0.,0.,141.3)) ;
#12079=CARTESIAN_POINT('',(-14.6232691283,-1.5,144.2)) ;
#12080=CARTESIAN_POINT('',(-14.6232691283,-1.5,130.439999998)) ;
#12081=CARTESIAN_POINT('Origin',(0.,0.,144.2)) ;
#12082=CARTESIAN_POINT('Origin',(-14.6232691283,-1.5,144.2)) ;
#12083=CARTESIAN_POINT('',(-13.4661044845,-1.5,141.3)) ;
#12084=CARTESIAN_POINT('',(-13.4661044845,-1.5,144.2)) ;
#12085=CARTESIAN_POINT('Origin',(0.,0.,130.439999998)) ;
#12086=CARTESIAN_POINT('',(-1.5,-7.2463784058,144.2)) ;
#12087=CARTESIAN_POINT('',(-1.5,-7.2463784058,141.3)) ;
#12088=CARTESIAN_POINT('',(-1.5,-7.2463784058,130.439999998)) ;
#12089=CARTESIAN_POINT('',(-7.2463784058,-1.5,144.2)) ;
#12090=CARTESIAN_POINT('Origin',(0.,0.,144.2)) ;
#12091=CARTESIAN_POINT('',(-7.2463784058,-1.5,141.3)) ;
#12092=CARTESIAN_POINT('',(-7.2463784058,-1.5,130.439999998)) ;
#12093=CARTESIAN_POINT('Origin',(0.,0.,141.3)) ;
#12094=CARTESIAN_POINT('Origin',(-1.5,-12.3089398406,144.2)) ;
#12095=CARTESIAN_POINT('',(-1.5,-9.58331884057,141.3)) ;
#12096=CARTESIAN_POINT('',(-1.5,-8.41484862318,141.3)) ;
#12097=CARTESIAN_POINT('',(-1.5,-9.58331884057,144.2)) ;
#12098=CARTESIAN_POINT('',(-1.5,-9.58331884057,142.75)) ;
#12099=CARTESIAN_POINT('',(-1.5,-8.41484862318,144.2)) ;
#12100=CARTESIAN_POINT('Origin',(0.,0.,130.439999998)) ;
#12101=CARTESIAN_POINT('',(-9.58331884057,-1.5,141.3)) ;
#12102=CARTESIAN_POINT('Origin',(0.,0.,141.3)) ;
#12103=CARTESIAN_POINT('',(-9.58331884057,-1.5,144.2)) ;
#12104=CARTESIAN_POINT('',(-9.58331884057,-1.5,130.439999998)) ;
#12105=CARTESIAN_POINT('Origin',(0.,0.,144.2)) ;
#12106=CARTESIAN_POINT('Origin',(-14.6232691283,-1.5,144.2)) ;
#12107=CARTESIAN_POINT('',(-8.41484862318,-1.5,141.3)) ;
#12108=CARTESIAN_POINT('',(-8.41484862318,-1.5,144.2)) ;
#12109=CARTESIAN_POINT('Origin',(0.,0.,130.439999998)) ;
#12110=CARTESIAN_POINT('',(-12.3089398406,1.5,144.2)) ;
#12111=CARTESIAN_POINT('',(-12.3089398406,1.5,141.3)) ;
#12112=CARTESIAN_POINT('',(-12.3089398406,1.5,130.439999998)) ;
#12113=CARTESIAN_POINT('',(-1.5,12.3089398406,144.2)) ;
#12114=CARTESIAN_POINT('Origin',(0.,0.,144.2)) ;
#12115=CARTESIAN_POINT('',(-1.5,12.3089398406,141.3)) ;
#12116=CARTESIAN_POINT('',(-1.5,12.3089398406,130.439999998)) ;
#12117=CARTESIAN_POINT('Origin',(0.,0.,141.3)) ;
#12118=CARTESIAN_POINT('Origin',(-14.6232691283,1.5,144.2)) ;
#12119=CARTESIAN_POINT('',(-14.6232691283,1.5,144.2)) ;
#12120=CARTESIAN_POINT('',(-14.6232691283,1.5,141.3)) ;
#12121=CARTESIAN_POINT('',(-14.6232691283,1.5,142.75)) ;
#12122=CARTESIAN_POINT('',(-13.4661044845,1.5,144.2)) ;
#12123=CARTESIAN_POINT('',(-13.4661044845,1.5,141.3)) ;
#12124=CARTESIAN_POINT('Origin',(0.,0.,130.439999998)) ;
#12125=CARTESIAN_POINT('',(-1.5,14.6232691283,141.3)) ;
#12126=CARTESIAN_POINT('Origin',(0.,0.,141.3)) ;
#12127=CARTESIAN_POINT('',(-1.5,14.6232691283,144.2)) ;
#12128=CARTESIAN_POINT('',(-1.5,14.6232691283,130.439999998)) ;
#12129=CARTESIAN_POINT('Origin',(0.,0.,144.2)) ;
#12130=CARTESIAN_POINT('Origin',(-1.5,-12.3089398406,144.2)) ;
#12131=CARTESIAN_POINT('',(-1.5,13.4661044845,141.3)) ;
#12132=CARTESIAN_POINT('',(-1.5,13.4661044845,144.2)) ;
#12133=CARTESIAN_POINT('Origin',(-14.6232691283,1.5,144.2)) ;
#12134=CARTESIAN_POINT('',(12.3089398406,1.5,144.2)) ;
#12135=CARTESIAN_POINT('',(12.3089398406,1.5,141.3)) ;
#12136=CARTESIAN_POINT('',(12.3089398406,1.5,142.75)) ;
#12137=CARTESIAN_POINT('',(14.6232691283,1.5,144.2)) ;
#12138=CARTESIAN_POINT('',(13.4661044845,1.5,144.2)) ;
#12139=CARTESIAN_POINT('',(14.6232691283,1.5,141.3)) ;
#12140=CARTESIAN_POINT('',(14.6232691283,1.5,142.75)) ;
#12141=CARTESIAN_POINT('',(13.4661044845,1.5,141.3)) ;
#12142=CARTESIAN_POINT('Origin',(0.,0.,130.439999998)) ;
#12143=CARTESIAN_POINT('',(1.5,12.3089398406,144.2)) ;
#12144=CARTESIAN_POINT('',(1.5,12.3089398406,141.3)) ;
#12145=CARTESIAN_POINT('',(1.5,12.3089398406,130.439999998)) ;
#12146=CARTESIAN_POINT('Origin',(0.,0.,144.2)) ;
#12147=CARTESIAN_POINT('Origin',(0.,0.,141.3)) ;
#12148=CARTESIAN_POINT('Origin',(1.5,14.6232691283,144.2)) ;
#12149=CARTESIAN_POINT('',(1.5,14.6232691283,144.2)) ;
#12150=CARTESIAN_POINT('',(1.5,14.6232691283,141.3)) ;
#12151=CARTESIAN_POINT('',(1.5,14.6232691283,142.75)) ;
#12152=CARTESIAN_POINT('',(1.5,13.4661044845,144.2)) ;
#12153=CARTESIAN_POINT('',(1.5,13.4661044845,141.3)) ;
#12154=CARTESIAN_POINT('Origin',(0.,0.,130.439999998)) ;
#12155=CARTESIAN_POINT('Origin',(0.,0.,141.3)) ;
#12156=CARTESIAN_POINT('Origin',(0.,0.,144.2)) ;
#12157=CARTESIAN_POINT('Origin',(-14.6232691283,-1.5,144.2)) ;
#12158=CARTESIAN_POINT('',(7.2463784058,-1.5,141.3)) ;
#12159=CARTESIAN_POINT('',(9.58331884057,-1.5,141.3)) ;
#12160=CARTESIAN_POINT('',(8.41484862318,-1.5,141.3)) ;
#12161=CARTESIAN_POINT('',(9.58331884057,-1.5,144.2)) ;
#12162=CARTESIAN_POINT('',(9.58331884057,-1.5,142.75)) ;
#12163=CARTESIAN_POINT('',(7.2463784058,-1.5,144.2)) ;
#12164=CARTESIAN_POINT('',(8.41484862318,-1.5,144.2)) ;
#12165=CARTESIAN_POINT('',(7.2463784058,-1.5,142.75)) ;
#12166=CARTESIAN_POINT('Origin',(0.,0.,130.439999998)) ;
#12167=CARTESIAN_POINT('',(1.5,-9.58331884057,141.3)) ;
#12168=CARTESIAN_POINT('Origin',(0.,0.,141.3)) ;
#12169=CARTESIAN_POINT('',(1.5,-9.58331884057,144.2)) ;
#12170=CARTESIAN_POINT('',(1.5,-9.58331884057,130.439999998)) ;
#12171=CARTESIAN_POINT('Origin',(0.,0.,144.2)) ;
#12172=CARTESIAN_POINT('Origin',(1.5,14.6232691283,144.2)) ;
#12173=CARTESIAN_POINT('',(1.5,-7.2463784058,144.2)) ;
#12174=CARTESIAN_POINT('',(1.5,-7.2463784058,141.3)) ;
#12175=CARTESIAN_POINT('',(1.5,-7.2463784058,142.75)) ;
#12176=CARTESIAN_POINT('',(1.5,-8.41484862318,144.2)) ;
#12177=CARTESIAN_POINT('',(1.5,-8.41484862318,141.3)) ;
#12178=CARTESIAN_POINT('Origin',(0.,0.,130.439999998)) ;
#12179=CARTESIAN_POINT('Origin',(0.,0.,144.2)) ;
#12180=CARTESIAN_POINT('Origin',(0.,0.,141.3)) ;
#12181=CARTESIAN_POINT('Origin',(1.5,14.6232691283,144.2)) ;
#12182=CARTESIAN_POINT('',(1.5,9.58331884057,144.2)) ;
#12183=CARTESIAN_POINT('',(1.5,9.58331884057,141.3)) ;
#12184=CARTESIAN_POINT('',(1.5,9.58331884057,142.75)) ;
#12185=CARTESIAN_POINT('',(1.5,7.2463784058,144.2)) ;
#12186=CARTESIAN_POINT('',(1.5,8.41484862318,144.2)) ;
#12187=CARTESIAN_POINT('',(1.5,7.2463784058,141.3)) ;
#12188=CARTESIAN_POINT('',(1.5,7.2463784058,142.75)) ;
#12189=CARTESIAN_POINT('',(1.5,8.41484862318,141.3)) ;
#12190=CARTESIAN_POINT('Origin',(0.,0.,130.439999998)) ;
#12191=CARTESIAN_POINT('',(9.58331884057,1.5,141.3)) ;
#12192=CARTESIAN_POINT('Origin',(0.,0.,141.3)) ;
#12193=CARTESIAN_POINT('',(9.58331884057,1.5,144.2)) ;
#12194=CARTESIAN_POINT('',(9.58331884057,1.5,130.439999998)) ;
#12195=CARTESIAN_POINT('Origin',(0.,0.,144.2)) ;
#12196=CARTESIAN_POINT('Origin',(-14.6232691283,1.5,144.2)) ;
#12197=CARTESIAN_POINT('',(7.2463784058,1.5,144.2)) ;
#12198=CARTESIAN_POINT('',(7.2463784058,1.5,141.3)) ;
#12199=CARTESIAN_POINT('',(7.2463784058,1.5,142.75)) ;
#12200=CARTESIAN_POINT('',(8.41484862318,1.5,144.2)) ;
#12201=CARTESIAN_POINT('',(8.41484862318,1.5,141.3)) ;
#12202=CARTESIAN_POINT('Origin',(0.,0.,130.439999998)) ;
#12203=CARTESIAN_POINT('Origin',(0.,0.,144.2)) ;
#12204=CARTESIAN_POINT('Origin',(0.,0.,141.3)) ;
#12205=CARTESIAN_POINT('Origin',(-1.5,-12.3089398406,144.2)) ;
#12206=CARTESIAN_POINT('',(-1.5,9.58331884057,141.3)) ;
#12207=CARTESIAN_POINT('',(-1.5,7.2463784058,141.3)) ;
#12208=CARTESIAN_POINT('',(-1.5,8.41484862318,141.3)) ;
#12209=CARTESIAN_POINT('',(-1.5,7.2463784058,144.2)) ;
#12210=CARTESIAN_POINT('',(-1.5,7.2463784058,142.75)) ;
#12211=CARTESIAN_POINT('',(-1.5,9.58331884057,144.2)) ;
#12212=CARTESIAN_POINT('',(-1.5,8.41484862318,144.2)) ;
#12213=CARTESIAN_POINT('',(-1.5,9.58331884057,142.75)) ;
#12214=CARTESIAN_POINT('Origin',(0.,0.,130.439999998)) ;
#12215=CARTESIAN_POINT('',(-7.2463784058,1.5,144.2)) ;
#12216=CARTESIAN_POINT('',(-7.2463784058,1.5,141.3)) ;
#12217=CARTESIAN_POINT('',(-7.2463784058,1.5,130.439999998)) ;
#12218=CARTESIAN_POINT('Origin',(0.,0.,144.2)) ;
#12219=CARTESIAN_POINT('Origin',(0.,0.,141.3)) ;
#12220=CARTESIAN_POINT('Origin',(-14.6232691283,1.5,144.2)) ;
#12221=CARTESIAN_POINT('',(-9.58331884057,1.5,144.2)) ;
#12222=CARTESIAN_POINT('',(-9.58331884057,1.5,141.3)) ;
#12223=CARTESIAN_POINT('',(-9.58331884057,1.5,142.75)) ;
#12224=CARTESIAN_POINT('',(-8.41484862318,1.5,144.2)) ;
#12225=CARTESIAN_POINT('',(-8.41484862318,1.5,141.3)) ;
#12226=CARTESIAN_POINT('Origin',(0.,0.,130.439999998)) ;
#12227=CARTESIAN_POINT('Origin',(0.,0.,141.3)) ;
#12228=CARTESIAN_POINT('Origin',(0.,0.,144.2)) ;
#12229=CARTESIAN_POINT('Origin',(-14.6232691283,-1.5,144.2)) ;
#12230=CARTESIAN_POINT('',(12.3089398406,-1.5,141.3)) ;
#12231=CARTESIAN_POINT('',(14.6232691283,-1.5,141.3)) ;
#12232=CARTESIAN_POINT('',(13.4661044845,-1.5,141.3)) ;
#12233=CARTESIAN_POINT('',(14.6232691283,-1.5,144.2)) ;
#12234=CARTESIAN_POINT('',(14.6232691283,-1.5,142.75)) ;
#12235=CARTESIAN_POINT('',(12.3089398406,-1.5,144.2)) ;
#12236=CARTESIAN_POINT('',(13.4661044845,-1.5,144.2)) ;
#12237=CARTESIAN_POINT('',(12.3089398406,-1.5,142.75)) ;
#12238=CARTESIAN_POINT('Origin',(0.,0.,130.439999998)) ;
#12239=CARTESIAN_POINT('',(1.5,-14.6232691283,141.3)) ;
#12240=CARTESIAN_POINT('Origin',(0.,0.,141.3)) ;
#12241=CARTESIAN_POINT('',(1.5,-14.6232691283,144.2)) ;
#12242=CARTESIAN_POINT('',(1.5,-14.6232691283,130.439999998)) ;
#12243=CARTESIAN_POINT('Origin',(0.,0.,144.2)) ;
#12244=CARTESIAN_POINT('Origin',(1.5,14.6232691283,144.2)) ;
#12245=CARTESIAN_POINT('',(1.5,-12.3089398406,144.2)) ;
#12246=CARTESIAN_POINT('',(1.5,-12.3089398406,141.3)) ;
#12247=CARTESIAN_POINT('',(1.5,-12.3089398406,142.75)) ;
#12248=CARTESIAN_POINT('',(1.5,-13.4661044845,144.2)) ;
#12249=CARTESIAN_POINT('',(1.5,-13.4661044845,141.3)) ;
#12250=CARTESIAN_POINT('Origin',(0.,0.,130.439999998)) ;
#12251=CARTESIAN_POINT('Origin',(0.,0.,144.2)) ;
#12252=CARTESIAN_POINT('Origin',(0.,0.,141.3)) ;
#12253=CARTESIAN_POINT('Origin',(0.,7.1054273576E-15,140.2)) ;
#12254=CARTESIAN_POINT('Origin',(0.,7.1054273576E-15,139.1)) ;
#12255=CARTESIAN_POINT('Origin',(0.,0.,140.2)) ;
#12256=CARTESIAN_POINT('Origin',(0.,0.,139.1)) ;
#12257=CARTESIAN_POINT('Origin',(0.,-3.52784468305E-12,141.3)) ;
#12258=CARTESIAN_POINT('Origin',(0.,0.,140.3)) ;
#12259=CARTESIAN_POINT('Origin',(0.,-25.,144.1)) ;
#12260=CARTESIAN_POINT('',(-2.51544272175,-26.2298568671,144.2)) ;
#12261=CARTESIAN_POINT('',(-2.45723117329304,-23.6576084919082,144.200000000002)) ;
#12262=CARTESIAN_POINT('Origin',(0.,-25.,144.2)) ;
#12263=CARTESIAN_POINT('',(2.51544272175,-26.2298568671,144.2)) ;
#12264=CARTESIAN_POINT('Ctrl Pts',(-2.51544272175672,-26.2298568671033,
144.2)) ;
#12265=CARTESIAN_POINT('Ctrl Pts',(-2.50680027005324,-26.2475333893208,
144.2)) ;
#12266=CARTESIAN_POINT('Ctrl Pts',(-2.49797002672654,-26.2651217394885,
144.199718757895)) ;
#12267=CARTESIAN_POINT('Ctrl Pts',(-2.37833537923512,-26.4972766533224,
144.192385578423)) ;
#12268=CARTESIAN_POINT('Ctrl Pts',(-2.24300310282228,-26.6911875549971,
144.145784256474)) ;
#12269=CARTESIAN_POINT('Ctrl Pts',(-1.88898180665551,-27.0894428011296,
143.98721671779)) ;
#12270=CARTESIAN_POINT('Ctrl Pts',(-1.64877360793947,-27.2842484628884,
143.852681685328)) ;
#12271=CARTESIAN_POINT('Ctrl Pts',(-1.1183576464604,-27.5843351802777,143.545257582706)) ;
#12272=CARTESIAN_POINT('Ctrl Pts',(-0.868883103158393,-27.6709706828989,
143.39696325339)) ;
#12273=CARTESIAN_POINT('Ctrl Pts',(-0.484562745701299,-27.7632226317754,
143.201577325697)) ;
#12274=CARTESIAN_POINT('Ctrl Pts',(-0.305793659353828,-27.788980090451,
143.121283953976)) ;
#12275=CARTESIAN_POINT('Ctrl Pts',(-0.101135302757054,-27.7982956567318,
143.090547872392)) ;
#12276=CARTESIAN_POINT('Ctrl Pts',(-0.0752436403656064,-27.7991071634455,
143.087813318513)) ;
#12277=CARTESIAN_POINT('Ctrl Pts',(-0.0398711158979192,-27.7997327010551,
143.085702521145)) ;
#12278=CARTESIAN_POINT('Ctrl Pts',(-0.0303643459146114,-27.799851098454,
143.08530176708)) ;
#12279=CARTESIAN_POINT('Ctrl Pts',(-0.0152865707782385,-27.7999640496678,
143.084919345159)) ;
#12280=CARTESIAN_POINT('Ctrl Pts',(-0.00967725965468007,-27.7999887480387,
143.084835652304)) ;
#12281=CARTESIAN_POINT('Ctrl Pts',(0.00183240768707374,-27.8000057743921,
143.084777964861)) ;
#12282=CARTESIAN_POINT('Ctrl Pts',(0.00772238672552688,-27.7999953807962,
143.084813192188)) ;
#12283=CARTESIAN_POINT('Ctrl Pts',(0.0213621632658133,-27.7999294545034,
143.085036496662)) ;
#12284=CARTESIAN_POINT('Ctrl Pts',(0.0290762552063979,-27.7998593663311,
143.085273870456)) ;
#12285=CARTESIAN_POINT('Ctrl Pts',(0.0535771921206085,-27.7995383345268,
143.086359150511)) ;
#12286=CARTESIAN_POINT('Ctrl Pts',(0.0701739806097318,-27.7991683272186,
143.087608442126)) ;
#12287=CARTESIAN_POINT('Ctrl Pts',(0.176346596798053,-27.7958857198553,
143.098593359858)) ;
#12288=CARTESIAN_POINT('Ctrl Pts',(0.281600510548293,-27.7889863704116,
143.124004371605)) ;
#12289=CARTESIAN_POINT('Ctrl Pts',(0.5673448927281,-27.746336371669,143.238520660015)) ;
#12290=CARTESIAN_POINT('Ctrl Pts',(0.733807526533163,-27.7083090209718,
143.326771017972)) ;
#12291=CARTESIAN_POINT('Ctrl Pts',(1.23380805912857,-27.537167755989,143.607475636533)) ;
#12292=CARTESIAN_POINT('Ctrl Pts',(1.56145101787667,-27.3567572246986,143.808570612768)) ;
#12293=CARTESIAN_POINT('Ctrl Pts',(2.07742533390529,-26.9008360197354,144.078456726255)) ;
#12294=CARTESIAN_POINT('Ctrl Pts',(2.25633674761856,-26.6794743095826,144.155188752781)) ;
#12295=CARTESIAN_POINT('Ctrl Pts',(2.43874719860503,-26.3782715768778,144.194978408393)) ;
#12296=CARTESIAN_POINT('Ctrl Pts',(2.47891544276577,-26.3045666000333,144.200000000002)) ;
#12297=CARTESIAN_POINT('Ctrl Pts',(2.51544272175672,-26.2298568671033,144.2)) ;
#12298=CARTESIAN_POINT('Origin',(0.,-25.,144.2)) ;
#12299=CARTESIAN_POINT('',(-2.45723117329304,-23.6576084919082,144.1)) ;
#12300=CARTESIAN_POINT('Origin',(0.,0.,139.1)) ;
#12301=CARTESIAN_POINT('',(21.6872098018009,10.950431579183,139.1)) ;
#12302=CARTESIAN_POINT('Origin',(21.6506350946,12.5,139.1)) ;
#12303=CARTESIAN_POINT('Origin',(0.,0.,139.1)) ;
#12304=CARTESIAN_POINT('',(-20.3269568308709,13.3064588359805,139.1)) ;
#12305=CARTESIAN_POINT('Origin',(-21.6506350946,12.5,139.1)) ;
#12306=CARTESIAN_POINT('Origin',(0.,-26.3501962679,144.2)) ;
#12307=CARTESIAN_POINT('',(-21.4580010236,15.2933657325,144.2)) ;
#12308=CARTESIAN_POINT('',(-19.2594743601216,13.9568288649971,144.200000000001)) ;
#12309=CARTESIAN_POINT('Origin',(-21.6506350946,12.5,144.2)) ;
#12310=CARTESIAN_POINT('',(-23.9734437454,10.9364911348,144.2)) ;
#12311=CARTESIAN_POINT('Origin',(-21.6506350946,12.5,144.2)) ;
#12312=CARTESIAN_POINT('Origin',(0.,0.,144.2)) ;
#12313=CARTESIAN_POINT('',(23.9734437455,10.9364911346,144.2)) ;
#12314=CARTESIAN_POINT('Origin',(0.,0.,144.2)) ;
#12315=CARTESIAN_POINT('',(21.7167055334145,9.7007796269113,144.200000000001)) ;
#12316=CARTESIAN_POINT('Origin',(21.6506350946,12.5,144.2)) ;
#12317=CARTESIAN_POINT('',(21.4580010237,15.2933657324,144.2)) ;
#12318=CARTESIAN_POINT('Origin',(21.6506350946,12.5,144.2)) ;
#12319=CARTESIAN_POINT('',(12.6329570380645,23.1244727470978,144.2)) ;
#12320=CARTESIAN_POINT('Origin',(0.,0.,144.2)) ;
#12321=CARTESIAN_POINT('Origin',(0.,0.,144.2)) ;
#12322=CARTESIAN_POINT('Origin',(0.,0.,142.7)) ;
#12323=CARTESIAN_POINT('Origin',(12.6329570380645,23.1244727470978,142.7)) ;
#12324=CARTESIAN_POINT('Ctrl Pts',(21.4580010237027,15.2933657323611,144.2)) ;
#12325=CARTESIAN_POINT('Ctrl Pts',(21.5409651897478,15.299087047282,144.2)) ;
#12326=CARTESIAN_POINT('Ctrl Pts',(21.6248796940807,15.3011528158356,144.194978408399)) ;
#12327=CARTESIAN_POINT('Ctrl Pts',(21.9769341376897,15.2937820977436,144.155188752827)) ;
#12328=CARTESIAN_POINT('Ctrl Pts',(22.2580947089449,15.2495211235406,144.078456726328)) ;
#12329=CARTESIAN_POINT('Ctrl Pts',(22.9109212125779,15.0306348607089,143.808570612899)) ;
#12330=CARTESIAN_POINT('Ctrl Pts',(23.230982795189,14.8370930007306,143.607475636674)) ;
#12331=CARTESIAN_POINT('Ctrl Pts',(23.6291957446838,14.4896504700656,143.326771018074)) ;
#12332=CARTESIAN_POINT('Ctrl Pts',(23.7453597133601,14.3645032757347,143.238520660095)) ;
#12333=CARTESIAN_POINT('Ctrl Pts',(23.9251678868797,14.1383663811055,143.124004371652)) ;
#12334=CARTESIAN_POINT('Ctrl Pts',(23.9837698556499,14.0506634926615,143.098593359902)) ;
#12335=CARTESIAN_POINT('Ctrl Pts',(24.0396989851174,13.9603566135313,143.087608442164)) ;
#12336=CARTESIAN_POINT('Ctrl Pts',(24.0483178150953,13.946168376725,143.086359150548)) ;
#12337=CARTESIAN_POINT('Ctrl Pts',(24.0608463052552,13.9251104588349,143.085273870492)) ;
#12338=CARTESIAN_POINT('Ctrl Pts',(24.0647640493649,13.9184649033307,143.085036496698)) ;
#12339=CARTESIAN_POINT('Ctrl Pts',(24.0716410314813,13.9066854734882,143.084813192224)) ;
#12340=CARTESIAN_POINT('Ctrl Pts',(24.074595022119,13.9015897988103,143.084777964896)) ;
#12341=CARTESIAN_POINT('Ctrl Pts',(24.0803351105353,13.8916136213267,143.08483565234)) ;
#12342=CARTESIAN_POINT('Ctrl Pts',(24.0831183766799,13.8867434662114,143.084919345194)) ;
#12343=CARTESIAN_POINT('Ctrl Pts',(24.0905594456277,13.8736292543037,143.085301767116)) ;
#12344=CARTESIAN_POINT('Ctrl Pts',(24.0952102954634,13.8653369512921,143.08570252118)) ;
#12345=CARTESIAN_POINT('Ctrl Pts',(24.1123548262279,13.834390677718,143.087813318547)) ;
#12346=CARTESIAN_POINT('Ctrl Pts',(24.124597871987,13.811562086998,143.090547872423)) ;
#12347=CARTESIAN_POINT('Ctrl Pts',(24.218859533259,13.6296649679125,143.121283953996)) ;
#12348=CARTESIAN_POINT('Ctrl Pts',(24.285937462891,13.461967668342,143.201577325746)) ;
#12349=CARTESIAN_POINT('Ctrl Pts',(24.3982051103286,13.0830105012164,143.396963253395)) ;
#12350=CARTESIAN_POINT('Ctrl Pts',(24.4479138358381,12.823641457819,143.545257582702)) ;
#12351=CARTESIAN_POINT('Ctrl Pts',(24.4532390959926,12.2142444019233,143.852681685317)) ;
#12352=CARTESIAN_POINT('Ctrl Pts',(24.4046365434684,11.9088151687524,143.98721671778)) ;
#12353=CARTESIAN_POINT('Ctrl Pts',(24.2367480312154,11.403096109715,144.145784256471)) ;
#12354=CARTESIAN_POINT('Ctrl Pts',(24.1364824025005,11.1889394695486,144.192385578421)) ;
#12355=CARTESIAN_POINT('Ctrl Pts',(23.9952476732394,10.9692553687052,144.199718757896)) ;
#12356=CARTESIAN_POINT('Ctrl Pts',(23.9844308368281,10.9528139785505,144.200000000001)) ;
#12357=CARTESIAN_POINT('Ctrl Pts',(23.9734437453696,10.9364911346878,144.2)) ;
#12358=CARTESIAN_POINT('Ctrl Pts',(-23.9734437454311,10.9364911347791,144.2)) ;
#12359=CARTESIAN_POINT('Ctrl Pts',(-24.019880632519,11.0054795527183,144.2)) ;
#12360=CARTESIAN_POINT('Ctrl Pts',(-24.0636268927324,11.0771187609412,144.1949784084)) ;
#12361=CARTESIAN_POINT('Ctrl Pts',(-24.2332708854233,11.385692211663,144.15518875283)) ;
#12362=CARTESIAN_POINT('Ctrl Pts',(-24.335520042997,11.6513148960117,144.078456726333)) ;
#12363=CARTESIAN_POINT('Ctrl Pts',(-24.472372230663,12.3261223638347,143.808570612907)) ;
#12364=CARTESIAN_POINT('Ctrl Pts',(-24.4647908545363,12.7000747551423,143.607475636683)) ;
#12365=CARTESIAN_POINT('Ctrl Pts',(-24.3630032713721,13.2186585508609,143.326771018079)) ;
#12366=CARTESIAN_POINT('Ctrl Pts',(-24.3127046062076,13.3818330959064,143.238520660098)) ;
#12367=CARTESIAN_POINT('Ctrl Pts',(-24.2067683974841,13.6506199893009,143.124004371653)) ;
#12368=CARTESIAN_POINT('Ctrl Pts',(-24.160116452491,13.7452222271909,143.098593359902)) ;
#12369=CARTESIAN_POINT('Ctrl Pts',(-24.1098729657611,13.8388117136872,143.087608442164)) ;
#12370=CARTESIAN_POINT('Ctrl Pts',(-24.1018950072409,13.8533699578019,143.086359150548)) ;
#12371=CARTESIAN_POINT('Ctrl Pts',(-24.0899225604786,13.8747489074942,143.085273870492)) ;
#12372=CARTESIAN_POINT('Ctrl Pts',(-24.0861262126438,13.881464551172,143.085036496698)) ;
#12373=CARTESIAN_POINT('Ctrl Pts',(-24.079363418216,13.8933099073079,143.084813192224)) ;
#12374=CARTESIAN_POINT('Ctrl Pts',(-24.0764274298142,13.8984159755821,143.084777964896)) ;
#12375=CARTESIAN_POINT('Ctrl Pts',(-24.0706578508874,13.9083751267149,143.08483565234)) ;
#12376=CARTESIAN_POINT('Ctrl Pts',(-24.0678318059082,13.9132205834614,143.084919345195)) ;
#12377=CARTESIAN_POINT('Ctrl Pts',(-24.0601950997221,13.9262218441508,143.085301767116)) ;
#12378=CARTESIAN_POINT('Ctrl Pts',(-24.0553391795764,13.9343957497629,143.08570252118)) ;
#12379=CARTESIAN_POINT('Ctrl Pts',(-24.0371111858904,13.9647164857289,143.087813318547)) ;
#12380=CARTESIAN_POINT('Ctrl Pts',(-24.0234625692737,13.9867335697361,143.090547872423)) ;
#12381=CARTESIAN_POINT('Ctrl Pts',(-23.9130658739086,14.15931512254,143.121283953996)) ;
#12382=CARTESIAN_POINT('Ctrl Pts',(-23.8013747171509,14.3012549634204,143.201577325744)) ;
#12383=CARTESIAN_POINT('Ctrl Pts',(-23.5293220071935,14.5879601816862,143.396963253393)) ;
#12384=CARTESIAN_POINT('Ctrl Pts',(-23.3295561894133,14.7606937224659,143.545257582698)) ;
#12385=CARTESIAN_POINT('Ctrl Pts',(-22.8044654880936,15.070004060989,143.852681685313)) ;
#12386=CARTESIAN_POINT('Ctrl Pts',(-22.5156547368479,15.1806276324019,143.987216717778)) ;
#12387=CARTESIAN_POINT('Ctrl Pts',(-21.9937449284149,15.2880914453061,144.145784256469)) ;
#12388=CARTESIAN_POINT('Ctrl Pts',(-21.7581470232848,15.308337183797,144.19238557842)) ;
#12389=CARTESIAN_POINT('Ctrl Pts',(-21.4972776465203,15.2958663707821,144.199718757896)) ;
#12390=CARTESIAN_POINT('Ctrl Pts',(-21.4776305667768,15.2947194107393,144.200000000001)) ;
#12391=CARTESIAN_POINT('Ctrl Pts',(-21.45800102361,15.2933657323548,144.2)) ;
#12392=CARTESIAN_POINT('Origin',(1.55,-25.,142.2)) ;
#12393=CARTESIAN_POINT('',(21.7167055334145,9.7007796269113,142.2)) ;
#12394=CARTESIAN_POINT('Origin',(21.6506350946,12.5,142.2)) ;
#12395=CARTESIAN_POINT('',(21.6872098018009,10.950431579183,142.2)) ;
#12396=CARTESIAN_POINT('Origin',(21.6506350946,12.5,142.2)) ;
#12397=CARTESIAN_POINT('Origin',(21.6506350946,12.5,144.1)) ;
#12398=CARTESIAN_POINT('',(21.7167055334145,9.7007796269113,144.1)) ;
#12399=CARTESIAN_POINT('Origin',(21.6506350946,12.5,144.1)) ;
#12400=CARTESIAN_POINT('',(21.6872098018009,10.950431579183,144.1)) ;
#12401=CARTESIAN_POINT('Origin',(1.55,-25.,142.2)) ;
#12402=CARTESIAN_POINT('',(-19.2594743601216,13.9568288649971,142.2)) ;
#12403=CARTESIAN_POINT('Origin',(-21.6506350946,12.5,142.2)) ;
#12404=CARTESIAN_POINT('',(-20.3269568308709,13.3064588359805,142.2)) ;
#12405=CARTESIAN_POINT('Origin',(-21.6506350946,12.5,142.2)) ;
#12406=CARTESIAN_POINT('Origin',(-21.6506350946,12.5,144.1)) ;
#12407=CARTESIAN_POINT('',(-19.2594743601216,13.9568288649971,144.1)) ;
#12408=CARTESIAN_POINT('Origin',(-21.6506350946,12.5,144.1)) ;
#12409=CARTESIAN_POINT('',(-20.3269568308709,13.3064588359805,144.1)) ;
#13480=UNCERTAINTY_MEASURE_WITH_UNIT(LENGTH_MEASURE(0.01),#13511,
'DISTANCE_ACCURACY_VALUE',
'Maximum model space distance between geometric entities at asserted c
onnectivities') ;
#13493=UNCERTAINTY_MEASURE_WITH_UNIT(LENGTH_MEASURE(0.01),#13511,
'DISTANCE_ACCURACY_VALUE',
'Maximum model space distance between geometric entities at asserted c
onnectivities') ;
#13497=(
GEOMETRIC_REPRESENTATION_CONTEXT(3)
GLOBAL_UNCERTAINTY_ASSIGNED_CONTEXT((#13480))
GLOBAL_UNIT_ASSIGNED_CONTEXT((#13511,#13513,#13514))
REPRESENTATION_CONTEXT('','3D')
) ;
#13510=(
GEOMETRIC_REPRESENTATION_CONTEXT(3)
GLOBAL_UNCERTAINTY_ASSIGNED_CONTEXT((#13493))
GLOBAL_UNIT_ASSIGNED_CONTEXT((#13511,#13513,#13514))
REPRESENTATION_CONTEXT('','3D')
) ;
#13511=(
LENGTH_UNIT()
NAMED_UNIT(*)
SI_UNIT(.MILLI.,.METRE.)
) ;
#13513=(
NAMED_UNIT(*)
PLANE_ANGLE_UNIT()
SI_UNIT($,.RADIAN.)
) ;
#13514=(
NAMED_UNIT(*)
SI_UNIT($,.STERADIAN.)
SOLID_ANGLE_UNIT()
) ;
#13518=SHAPE_DEFINITION_REPRESENTATION(#13534,#13565) ;
#13534=PRODUCT_DEFINITION_SHAPE('',$,#13582) ;
#13565=SHAPE_REPRESENTATION('',(#7893),#13497) ;
#13578=PRODUCT_DEFINITION_CONTEXT('part definition',#13628,'design') ;
#13582=PRODUCT_DEFINITION('Motor_Housing','Motor_Housing',#13598,#13578) ;
#13598=PRODUCT_DEFINITION_FORMATION('',$,#13633) ;
#13628=APPLICATION_CONTEXT(
'Core Data for Automotive Mechanical Design Process') ;
#13629=PRODUCT_CONTEXT('part definition',#13628,'mechanical') ;
#13633=PRODUCT('Motor_Housing','Motor_Housing',$,(#13629)) ;
#13649=PRESENTATION_STYLE_ASSIGNMENT((#13654)) ;
#13654=SURFACE_STYLE_USAGE(.BOTH.,#13659) ;
#13659=SURFACE_SIDE_STYLE('',(#13664)) ;
#13664=SURFACE_STYLE_FILL_AREA(#13669) ;
#13669=FILL_AREA_STYLE('Opaque(50,50,50)',(#13674)) ;
#13674=FILL_AREA_STYLE_COLOUR('Opaque(50,50,50)',#13679) ;
#13679=COLOUR_RGB('Opaque(50,50,50)', 0.31764706, 0.68627451, 0.89019608) ;
ENDSEC;
END-ISO-10303-21;
